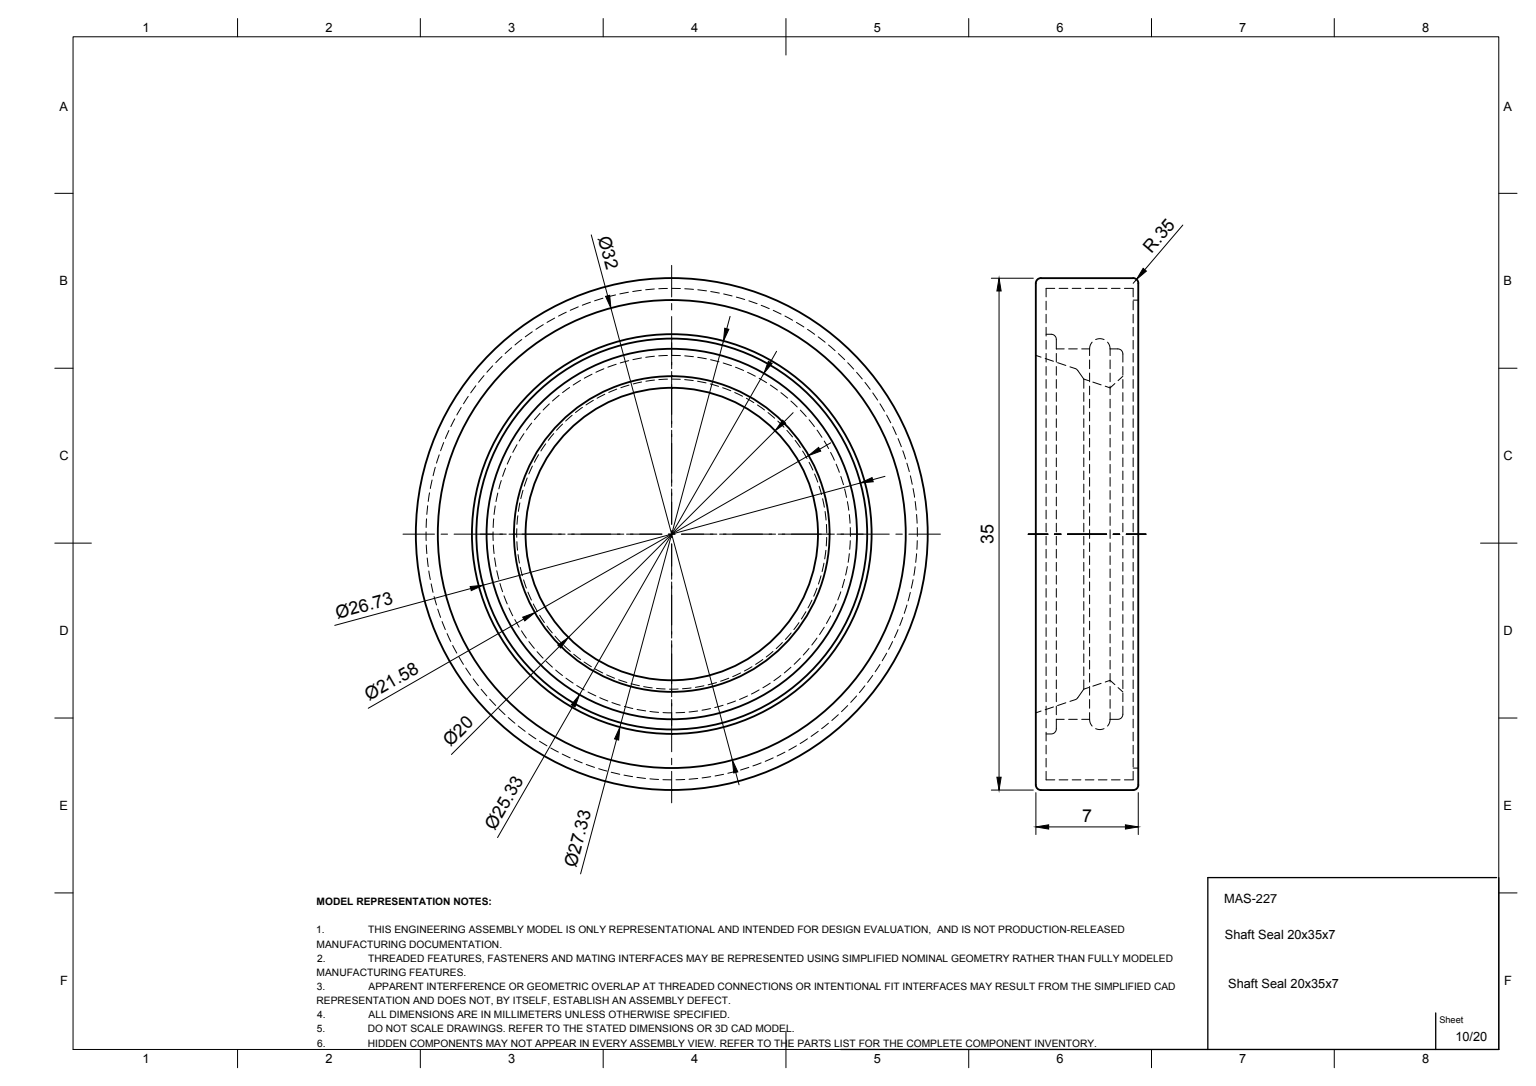
ISO-10303-21;
HEADER;
FILE_DESCRIPTION (('STEP AP214'),
    '1' );
FILE_NAME ( 'Shaft Seal 20x35x7.step', '2026-10-06T08:24:41', ( '' ), ( '' ), 'STEP AP214', 'Unspecified', '' );
FILE_SCHEMA (( 'AUTOMOTIVE_DESIGN' ));
ENDSEC;
DATA;
#55=EDGE_CURVE ( 'NONE', #27011, #13237, #9086, .T. ) ;
#110=CIRCLE ( 'NONE', #17215, 0.4848217985909654137 ) ;
#132=CIRCLE ( 'NONE', #21747, 0.6299212598425196763 ) ;
#156=ORIENTED_EDGE ( 'NONE', *, *, #27125, .T. ) ;
#161=CARTESIAN_POINT ( 'NONE',  ( 0.000000000000000000, 0.000000000000000000, -0.1033464566929133965 ) ) ;
#196=CARTESIAN_POINT ( 'NONE',  ( -0.6751968503937006982, 0.000000000000000000, -0.2618110236220472231 ) ) ;
#313=DIRECTION ( 'NONE',  ( -1.000000000000000000, 0.000000000000000000, 0.000000000000000000 ) ) ;
#322=FACE_OUTER_BOUND ( 'NONE', #12534, .T. ) ;
#345=ORIENTED_EDGE ( 'NONE', *, *, #3993, .T. ) ;
#363=DIRECTION ( 'NONE',  ( 0.000000000000000000, 0.000000000000000000, -1.000000000000000000 ) ) ;
#374=AXIS2_PLACEMENT_3D ( 'NONE', #10936, #6568, #8678 ) ;
#398=DIRECTION ( 'NONE',  ( -1.000000000000000000, 0.000000000000000000, 0.000000000000000000 ) ) ;
#418=DIRECTION ( 'NONE',  ( -1.000000000000000000, 0.000000000000000000, 0.000000000000000000 ) ) ;
#425=AXIS2_PLACEMENT_3D ( 'NONE', #17792, #8636, #2410 ) ;
#446=FACE_BOUND ( 'NONE', #5587, .T. ) ;
#490=CARTESIAN_POINT ( 'NONE',  ( -0.6614173228346456046, 0.000000000000000000, -0.2480314960629921295 ) ) ;
#495=DIRECTION ( 'NONE',  ( 0.000000000000000000, 0.000000000000000000, 1.000000000000000000 ) ) ;
#507=DIRECTION ( 'NONE',  ( 0.000000000000000000, 0.000000000000000000, -1.000000000000000000 ) ) ;
#540=EDGE_LOOP ( 'NONE', ( #5491, #24841, #13223, #6608 ) ) ;
#544=EDGE_CURVE ( 'NONE', #25079, #10563, #9634, .T. ) ;
#545=CIRCLE ( 'NONE', #13618, 0.01377952755905510404 ) ;
#623=CARTESIAN_POINT ( 'NONE',  ( 0.000000000000000000, 0.000000000000000000, -0.05511811023622047168 ) ) ;
#825=EDGE_CURVE ( 'NONE', #24109, #24279, #17361, .T. ) ;
#839=ORIENTED_EDGE ( 'NONE', *, *, #24552, .T. ) ;
#850=AXIS2_PLACEMENT_3D ( 'NONE', #25833, #6763, #15396 ) ;
#877=AXIS2_PLACEMENT_3D ( 'NONE', #9629, #24334, #22215 ) ;
#909=AXIS2_PLACEMENT_3D ( 'NONE', #18396, #16022, #13901 ) ;
#932=CARTESIAN_POINT ( 'NONE',  ( 0.6751968503937006982, 8.353151887884997269E-17, -4.097771653543307347E-17 ) ) ;
#943=DIRECTION ( 'NONE',  ( 1.000000000000000000, 0.000000000000000000, 0.000000000000000000 ) ) ;
#1020=DIRECTION ( 'NONE',  ( -1.000000000000000000, 0.000000000000000000, 0.000000000000000000 ) ) ;
#1062=VECTOR ( 'NONE', #24990, 39.37007874015748143 ) ;
#1129=CARTESIAN_POINT ( 'NONE',  ( -0.5850448763834590338, 0.000000000000000000, -0.2755905511811023723 ) ) ;
#1147=ORIENTED_EDGE ( 'NONE', *, *, #20181, .T. ) ;
#1182=ADVANCED_FACE ( 'NONE', ( #9849 ), #22775, .T. ) ;
#1214=EDGE_LOOP ( 'NONE', ( #23740, #11327, #1147, #4046 ) ) ;
#1232=ORIENTED_EDGE ( 'NONE', *, *, #23960, .F. ) ;
#1257=CARTESIAN_POINT ( 'NONE',  ( -0.4173606904761050229, 0.000000000000000000, -0.1464516454673935042 ) ) ;
#1259=ORIENTED_EDGE ( 'NONE', *, *, #11342, .T. ) ;
#1336=( CONVERSION_BASED_UNIT ( 'INCH', #25059 ) LENGTH_UNIT ( ) NAMED_UNIT ( #10443 ) ) ;
#1337=VECTOR ( 'NONE', #1696, 39.37007874015748854 ) ;
#1355=DIRECTION ( 'NONE',  ( -1.000000000000000000, 0.000000000000000000, 0.000000000000000000 ) ) ;
#1357=ORIENTED_EDGE ( 'NONE', *, *, #3422, .F. ) ;
#1416=EDGE_LOOP ( 'NONE', ( #17196, #23650, #10052, #15549 ) ) ;
#1470=CARTESIAN_POINT ( 'NONE',  ( 0.4848217985909654137, 6.021729909607683004E-17, -0.04133858267716535029 ) ) ;
#1492=AXIS2_PLACEMENT_3D ( 'NONE', #22889, #26835, #7774 ) ;
#1536=AXIS2_PLACEMENT_3D ( 'NONE', #16554, #14463, #7522 ) ;
#1541=CIRCLE ( 'NONE', #24983, 0.6614173228346456046 ) ;
#1574=FACE_OUTER_BOUND ( 'NONE', #540, .T. ) ;
#1603=ORIENTED_EDGE ( 'NONE', *, *, #23444, .F. ) ;
#1619=CARTESIAN_POINT ( 'NONE',  ( 0.5379714048901780288, 6.588249590315613132E-17, -0.2480314960629921295 ) ) ;
#1641=CIRCLE ( 'NONE', #24186, 0.01377952755905510404 ) ;
#1646=LINE ( 'NONE', #27513, #5048 ) ;
#1678=CARTESIAN_POINT ( 'NONE',  ( 0.000000000000000000, 0.000000000000000000, -0.01377952755905511792 ) ) ;
#1696=DIRECTION ( 'NONE',  ( -0.6698894744055998718, 0.000000000000000000, 0.7424608353849979636 ) ) ;
#1697=CARTESIAN_POINT ( 'NONE',  ( 0.5241918773311228241, 6.419499047126015796E-17, -0.2342519685039370358 ) ) ;
#1735=VECTOR ( 'NONE', #24190, 39.37007874015748854 ) ;
#1792=DIRECTION ( 'NONE',  ( -1.000000000000000000, -1.224646799147356165E-16, 0.000000000000000000 ) ) ;
#1807=CARTESIAN_POINT ( 'NONE',  ( 0.6889763779527560139, 8.437527159479796553E-17, -0.2618110236220472231 ) ) ;
#1817=AXIS2_PLACEMENT_3D ( 'NONE', #6481, #17216, #21462 ) ;
#1838=FACE_OUTER_BOUND ( 'NONE', #26109, .T. ) ;
#1863=CIRCLE ( 'NONE', #3660, 0.4811133748141622202 ) ;
#1903=DIRECTION ( 'NONE',  ( 0.000000000000000000, 0.000000000000000000, -1.000000000000000000 ) ) ;
#1924=DIRECTION ( 'NONE',  ( -1.224646799147353207E-16, 1.000000000000000000, 0.000000000000000000 ) ) ;
#1925=DIRECTION ( 'NONE',  ( -1.000000000000000000, 0.000000000000000000, 0.000000000000000000 ) ) ;
#2015=CARTESIAN_POINT ( 'NONE',  ( -0.6299212598425196763, 0.000000000000000000, -4.370956692913385731E-17 ) ) ;
#2027=DIRECTION ( 'NONE',  ( 1.000000000000000000, 0.000000000000000000, 0.000000000000000000 ) ) ;
#2056=CARTESIAN_POINT ( 'NONE',  ( -0.4456396174367268093, -1.277930342114489576E-27, -0.1696422624804970747 ) ) ;
#2082=CARTESIAN_POINT ( 'NONE',  ( -0.6889763779527560139, 0.000000000000000000, -0.01377952755905511792 ) ) ;
#2174=CARTESIAN_POINT ( 'NONE',  ( 0.4986013261500205074, 6.106105181202481056E-17, -0.05511811023622047168 ) ) ;
#2177=LINE ( 'NONE', #19551, #13048 ) ;
#2184=FACE_BOUND ( 'NONE', #13764, .T. ) ;
#2223=VERTEX_POINT ( 'NONE', #14401 ) ;
#2240=CARTESIAN_POINT ( 'NONE',  ( -0.5996943638624113726, 0.000000000000000000, -0.2480314960629921295 ) ) ;
#2244=ORIENTED_EDGE ( 'NONE', *, *, #3504, .T. ) ;
#2262=CARTESIAN_POINT ( 'NONE',  ( 0.000000000000000000, 0.000000000000000000, -0.1309055118110236116 ) ) ;
#2267=CARTESIAN_POINT ( 'NONE',  ( 0.000000000000000000, 0.000000000000000000, -0.07578740157480315376 ) ) ;
#2276=ORIENTED_EDGE ( 'NONE', *, *, #7179, .T. ) ;
#2284=DIRECTION ( 'NONE',  ( 0.000000000000000000, 0.000000000000000000, -1.000000000000000000 ) ) ;
#2373=DIRECTION ( 'NONE',  ( 1.000000000000000000, 0.000000000000000000, 0.000000000000000000 ) ) ;
#2405=CARTESIAN_POINT ( 'NONE',  ( 0.000000000000000000, 0.000000000000000000, -0.2204724409448818867 ) ) ;
#2410=DIRECTION ( 'NONE',  ( 1.000000000000000000, 0.000000000000000000, 0.000000000000000000 ) ) ;
#2422=EDGE_CURVE ( 'NONE', #3726, #27011, #7034, .T. ) ;
#2429=DIRECTION ( 'NONE',  ( -1.000000000000000000, 0.000000000000000000, 0.000000000000000000 ) ) ;
#2432=EDGE_CURVE ( 'NONE', #12340, #4895, #14270, .T. ) ;
#2433=DIRECTION ( 'NONE',  ( -1.000000000000000000, 0.000000000000000000, 0.000000000000000000 ) ) ;
#2487=VERTEX_POINT ( 'NONE', #490 ) ;
#2548=ORIENTED_EDGE ( 'NONE', *, *, #8868, .F. ) ;
#2579=FACE_OUTER_BOUND ( 'NONE', #25724, .T. ) ;
#2580=EDGE_LOOP ( 'NONE', ( #27237, #13937 ) ) ;
#2585=DIRECTION ( 'NONE',  ( 0.000000000000000000, 0.000000000000000000, -1.000000000000000000 ) ) ;
#2604=ADVANCED_FACE ( 'NONE', ( #15156 ), #8024, .T. ) ;
#2633=EDGE_LOOP ( 'NONE', ( #23889, #12887 ) ) ;
#2685=ORIENTED_EDGE ( 'NONE', *, *, #23444, .T. ) ;
#2704=AXIS2_PLACEMENT_3D ( 'NONE', #14804, #21278, #1355 ) ;
#2729=EDGE_CURVE ( 'NONE', #12355, #25409, #17051, .T. ) ;
#2906=FACE_OUTER_BOUND ( 'NONE', #24076, .T. ) ;
#2916=DIRECTION ( 'NONE',  ( 0.000000000000000000, 0.000000000000000000, -1.000000000000000000 ) ) ;
#2923=CIRCLE ( 'NONE', #4729, 0.6614173228346456046 ) ;
#2962=DIRECTION ( 'NONE',  ( -1.000000000000000000, 0.000000000000000000, 0.000000000000000000 ) ) ;
#3008=EDGE_CURVE ( 'NONE', #23052, #25295, #24687, .T. ) ;
#3022=MANIFOLD_SOLID_BREP ( 'Shaft Seal 20x35x7', #25894 ) ;
#3050=DIRECTION ( 'NONE',  ( 1.000000000000000000, 0.000000000000000000, 0.000000000000000000 ) ) ;
#3097=ADVANCED_FACE ( 'NONE', ( #2906 ), #20667, .T. ) ;
#3143=AXIS2_PLACEMENT_3D ( 'NONE', #25557, #10283, #3501 ) ;
#3205=ADVANCED_FACE ( 'NONE', ( #15750 ), #24270, .T. ) ;
#3275=CARTESIAN_POINT ( 'NONE',  ( 0.3937007874015748254, -5.011764252456519698E-17, -0.07578740157480315376 ) ) ;
#3292=( NAMED_UNIT ( * ) PLANE_ANGLE_UNIT ( ) SI_UNIT ( $, .RADIAN. ) ) ;
#3307=DIRECTION ( 'NONE',  ( 0.000000000000000000, 0.000000000000000000, -1.000000000000000000 ) ) ;
#3366=DIRECTION ( 'NONE',  ( -1.000000000000000000, 0.000000000000000000, 0.000000000000000000 ) ) ;
#3382=CARTESIAN_POINT ( 'NONE',  ( 0.000000000000000000, 0.000000000000000000, -0.2204724409448818867 ) ) ;
#3422=EDGE_CURVE ( 'NONE', #18692, #19022, #26099, .T. ) ;
#3424=CARTESIAN_POINT ( 'NONE',  ( 0.000000000000000000, 0.000000000000000000, -0.2342519685039370358 ) ) ;
#3467=CARTESIAN_POINT ( 'NONE',  ( -0.6889763779527560139, 0.000000000000000000, -0.2618110236220472231 ) ) ;
#3501=DIRECTION ( 'NONE',  ( -1.000000000000000000, 0.000000000000000000, 0.000000000000000000 ) ) ;
#3504=EDGE_CURVE ( 'NONE', #23082, #16707, #15586, .T. ) ;
#3524=EDGE_CURVE ( 'NONE', #5922, #27503, #14854, .T. ) ;
#3548=ORIENTED_EDGE ( 'NONE', *, *, #19521, .F. ) ;
#3553=CARTESIAN_POINT ( 'NONE',  ( 0.000000000000000000, 0.000000000000000000, -0.01377952755905511792 ) ) ;
#3558=FACE_OUTER_BOUND ( 'NONE', #10210, .T. ) ;
#3565=CARTESIAN_POINT ( 'NONE',  ( 0.000000000000000000, 0.000000000000000000, -0.2342519685039370358 ) ) ;
#3570=AXIS2_PLACEMENT_3D ( 'NONE', #23741, #14865, #12984 ) ;
#3588=CIRCLE ( 'NONE', #23495, 0.6299212598425196763 ) ;
#3615=LINE ( 'NONE', #12246, #4669 ) ;
#3644=DIRECTION ( 'NONE',  ( 0.000000000000000000, 0.000000000000000000, 1.000000000000000000 ) ) ;
#3660=AXIS2_PLACEMENT_3D ( 'NONE', #26675, #26822, #22446 ) ;
#3665=DIRECTION ( 'NONE',  ( 0.000000000000000000, 0.000000000000000000, 1.000000000000000000 ) ) ;
#3726=VERTEX_POINT ( 'NONE', #24193 ) ;
#3780=ORIENTED_EDGE ( 'NONE', *, *, #20283, .F. ) ;
#3817=AXIS2_PLACEMENT_3D ( 'NONE', #5847, #27177, #7818 ) ;
#3880=AXIS2_PLACEMENT_3D ( 'NONE', #5456, #3307, #11949 ) ;
#3910=EDGE_LOOP ( 'NONE', ( #15781, #1259, #839, #24102 ) ) ;
#3930=CARTESIAN_POINT ( 'NONE',  ( 0.4055307389460929279, 4.966319214061935299E-17, -0.1111195235210984261 ) ) ;
#3978=CIRCLE ( 'NONE', #19758, 0.6889763779527560139 ) ;
#3989=CARTESIAN_POINT ( 'NONE',  ( 0.000000000000000000, 0.000000000000000000, -0.2618110236220472231 ) ) ;
#3993=EDGE_CURVE ( 'NONE', #3726, #15200, #17111, .T. ) ;
#3996=AXIS2_PLACEMENT_3D ( 'NONE', #161, #4361, #418 ) ;
#4046=ORIENTED_EDGE ( 'NONE', *, *, #6905, .F. ) ;
#4062=ORIENTED_EDGE ( 'NONE', *, *, #15737, .F. ) ;
#4084=CIRCLE ( 'NONE', #19402, 0.01377952755905510404 ) ;
#4138=DIRECTION ( 'NONE',  ( -1.000000000000000000, -1.224646799147356165E-16, 0.000000000000000000 ) ) ;
#4222=CARTESIAN_POINT ( 'NONE',  ( -0.4307823082429378392, 0.000000000000000000, -0.1559029880880275776 ) ) ;
#4226=LINE ( 'NONE', #26104, #11288 ) ;
#4256=DIRECTION ( 'NONE',  ( 0.000000000000000000, 0.000000000000000000, -1.000000000000000000 ) ) ;
#4283=LINE ( 'NONE', #9058, #23272 ) ;
#4287=TOROIDAL_SURFACE ( 'NONE', #7899, 0.6751968503937006982, 0.01377952755905511792 ) ;
#4290=EDGE_LOOP ( 'NONE', ( #7597, #11737 ) ) ;
#4345=ORIENTED_EDGE ( 'NONE', *, *, #19521, .T. ) ;
#4361=DIRECTION ( 'NONE',  ( 0.000000000000000000, 0.000000000000000000, -1.000000000000000000 ) ) ;
#4390=CARTESIAN_POINT ( 'NONE',  ( 0.6299212598425196763, 7.714310545810098438E-17, -0.01377952755905511792 ) ) ;
#4401=DIRECTION ( 'NONE',  ( -1.000000000000000000, 0.000000000000000000, 0.000000000000000000 ) ) ;
#4465=EDGE_CURVE ( 'NONE', #24279, #12499, #12727, .T. ) ;
#4470=AXIS2_PLACEMENT_3D ( 'NONE', #9684, #5310, #943 ) ;
#4476=EDGE_LOOP ( 'NONE', ( #27104, #19325, #20943, #13965 ) ) ;
#4480=CIRCLE ( 'NONE', #9406, 0.6751968503937006982 ) ;
#4510=CARTESIAN_POINT ( 'NONE',  ( 0.000000000000000000, 0.000000000000000000, -0.2342519685039370358 ) ) ;
#4538=CARTESIAN_POINT ( 'NONE',  ( 0.4173606904761050229, 5.111194336814911913E-17, -0.1464516454673935042 ) ) ;
#4552=VERTEX_POINT ( 'NONE', #2082 ) ;
#4573=EDGE_CURVE ( 'NONE', #16402, #11118, #26557, .T. ) ;
#4642=CARTESIAN_POINT ( 'NONE',  ( 0.6751968503937006982, 8.353151887884997269E-17, -0.2755905511811023723 ) ) ;
#4669=VECTOR ( 'NONE', #6048, 39.37007874015748143 ) ;
#4729=AXIS2_PLACEMENT_3D ( 'NONE', #14420, #9581, #12972 ) ;
#4743=CARTESIAN_POINT ( 'NONE',  ( 0.000000000000000000, 0.000000000000000000, -0.006889763779527558960 ) ) ;
#4786=EDGE_LOOP ( 'NONE', ( #13307, #18454, #15039, #24615 ) ) ;
#4863=EDGE_LOOP ( 'NONE', ( #16587, #345, #25002, #11154 ) ) ;
#4895=VERTEX_POINT ( 'NONE', #2174 ) ;
#4909=FACE_OUTER_BOUND ( 'NONE', #12771, .T. ) ;
#4947=FACE_OUTER_BOUND ( 'NONE', #10950, .T. ) ;
#5048=VECTOR ( 'NONE', #17907, 39.37007874015748143 ) ;
#5055=ORIENTED_EDGE ( 'NONE', *, *, #15114, .F. ) ;
#5144=ORIENTED_EDGE ( 'NONE', *, *, #2432, .T. ) ;
#5145=CIRCLE ( 'NONE', #3817, 0.5379714048901780288 ) ;
#5158=AXIS2_PLACEMENT_3D ( 'NONE', #4510, #15126, #12978 ) ;
#5229=CARTESIAN_POINT ( 'NONE',  ( 0.000000000000000000, 0.000000000000000000, 0.000000000000000000 ) ) ;
#5235=ORIENTED_EDGE ( 'NONE', *, *, #8944, .T. ) ;
#5239=ADVANCED_FACE ( 'NONE', ( #4947 ), #24748, .F. ) ;
#5281=DIRECTION ( 'NONE',  ( -1.000000000000000000, 0.000000000000000000, 0.000000000000000000 ) ) ;
#5293=ORIENTED_EDGE ( 'NONE', *, *, #21682, .F. ) ;
#5310=DIRECTION ( 'NONE',  ( 0.000000000000000000, 0.000000000000000000, 1.000000000000000000 ) ) ;
#5318=VECTOR ( 'NONE', #11192, 39.37007874015748143 ) ;
#5353=ADVANCED_FACE ( 'NONE', ( #6089, #12977 ), #14853, .T. ) ;
#5358=CARTESIAN_POINT ( 'NONE',  ( 0.000000000000000000, 0.000000000000000000, -0.05511811023622047168 ) ) ;
#5449=CARTESIAN_POINT ( 'NONE',  ( 0.000000000000000000, 0.000000000000000000, -0.04133858267716535029 ) ) ;
#5456=CARTESIAN_POINT ( 'NONE',  ( 0.000000000000000000, 0.000000000000000000, -0.2480314960629921295 ) ) ;
#5464=CARTESIAN_POINT ( 'NONE',  ( 0.000000000000000000, 0.000000000000000000, -0.2204724409448818867 ) ) ;
#5488=ADVANCED_FACE ( 'NONE', ( #4909 ), #13663, .F. ) ;
#5491=ORIENTED_EDGE ( 'NONE', *, *, #544, .T. ) ;
#5587=EDGE_LOOP ( 'NONE', ( #13267, #5293 ) ) ;
#5786=PRODUCT_DEFINITION_FORMATION_WITH_SPECIFIED_SOURCE ( 'ANY', '', #10231, .NOT_KNOWN. ) ;
#5809=DIRECTION ( 'NONE',  ( -1.000000000000000000, -1.224646799147356165E-16, 0.000000000000000000 ) ) ;
#5838=DIRECTION ( 'NONE',  ( 0.000000000000000000, 0.000000000000000000, -1.000000000000000000 ) ) ;
#5847=CARTESIAN_POINT ( 'NONE',  ( 0.000000000000000000, 0.000000000000000000, -0.2342519685039370358 ) ) ;
#5901=DIRECTION ( 'NONE',  ( -1.000000000000000000, 0.000000000000000000, 0.000000000000000000 ) ) ;
#5907=EDGE_CURVE ( 'NONE', #25295, #23039, #2177, .T. ) ;
#5922=VERTEX_POINT ( 'NONE', #1470 ) ;
#6048=DIRECTION ( 'NONE',  ( 0.000000000000000000, 0.000000000000000000, -1.000000000000000000 ) ) ;
#6055=PRODUCT_CONTEXT ( 'NONE', #6560, 'mechanical' ) ;
#6070=ORIENTED_EDGE ( 'NONE', *, *, #14605, .T. ) ;
#6072=CIRCLE ( 'NONE', #1536, 0.6751968503937006982 ) ;
#6089=FACE_BOUND ( 'NONE', #20083, .T. ) ;
#6103=CARTESIAN_POINT ( 'NONE',  ( 0.000000000000000000, 0.000000000000000000, -0.01377952755905511792 ) ) ;
#6125=CARTESIAN_POINT ( 'NONE',  ( -0.6751968503937006982, 0.000000000000000000, -4.097771653543307347E-17 ) ) ;
#6171=LINE ( 'NONE', #21406, #12454 ) ;
#6186=EDGE_CURVE ( 'NONE', #23082, #27011, #26137, .T. ) ;
#6232=CONICAL_SURFACE ( 'NONE', #374, 0.4626586504047134341, 0.3230892413134545116 ) ;
#6264=AXIS2_PLACEMENT_3D ( 'NONE', #12898, #21525, #2027 ) ;
#6273=DIRECTION ( 'NONE',  ( -1.000000000000000000, 0.000000000000000000, 0.000000000000000000 ) ) ;
#6282=PRODUCT_DEFINITION_CONTEXT ( 'detailed design', #13230, 'design' ) ;
#6313=DIRECTION ( 'NONE',  ( -1.000000000000000000, -1.224646799147356165E-16, 0.000000000000000000 ) ) ;
#6322=ORIENTED_EDGE ( 'NONE', *, *, #20618, .T. ) ;
#6362=CARTESIAN_POINT ( 'NONE',  ( -0.4092416079569000109, 0.000000000000000000, -0.05856299212598425896 ) ) ;
#6410=DIRECTION ( 'NONE',  ( 0.000000000000000000, 0.000000000000000000, -1.000000000000000000 ) ) ;
#6423=TOROIDAL_SURFACE ( 'NONE', #16342, 0.5241918773311228241, 0.01377952755905511792 ) ;
#6481=CARTESIAN_POINT ( 'NONE',  ( 0.000000000000000000, 0.000000000000000000, -4.097771653543307347E-17 ) ) ;
#6505=DIRECTION ( 'NONE',  ( 0.000000000000000000, 0.000000000000000000, -1.000000000000000000 ) ) ;
#6521=ADVANCED_FACE ( 'NONE', ( #8833 ), #25698, .F. ) ;
#6523=DIRECTION ( 'NONE',  ( 0.000000000000000000, 0.000000000000000000, -1.000000000000000000 ) ) ;
#6525=CIRCLE ( 'NONE', #19618, 0.6299212598425196763 ) ;
#6539=EDGE_LOOP ( 'NONE', ( #14520, #16363 ) ) ;
#6560=APPLICATION_CONTEXT ( 'automotive_design' ) ;
#6568=DIRECTION ( 'NONE',  ( 0.000000000000000000, 0.000000000000000000, -1.000000000000000000 ) ) ;
#6582=FACE_OUTER_BOUND ( 'NONE', #22443, .T. ) ;
#6608=ORIENTED_EDGE ( 'NONE', *, *, #8944, .F. ) ;
#6622=LINE ( 'NONE', #4222, #7707 ) ;
#6656=CARTESIAN_POINT ( 'NONE',  ( 0.6614173228346456046, 8.100026073100603114E-17, -0.01377952755905511792 ) ) ;
#6670=AXIS2_PLACEMENT_3D ( 'NONE', #21700, #1924, #6313 ) ;
#6687=DIRECTION ( 'NONE',  ( 0.000000000000000000, 0.000000000000000000, -1.000000000000000000 ) ) ;
#6741=FACE_OUTER_BOUND ( 'NONE', #22510, .T. ) ;
#6746=ORIENTED_EDGE ( 'NONE', *, *, #22676, .F. ) ;
#6763=DIRECTION ( 'NONE',  ( 0.000000000000000000, 0.000000000000000000, -1.000000000000000000 ) ) ;
#6765=ORIENTED_EDGE ( 'NONE', *, *, #13241, .T. ) ;
#6844=AXIS2_PLACEMENT_3D ( 'NONE', #15634, #7014, #398 ) ;
#6865=CARTESIAN_POINT ( 'NONE',  ( 0.4811133747915324332, 5.891939544654311124E-17, -0.2755905511811023723 ) ) ;
#6872=DIRECTION ( 'NONE',  ( 0.000000000000000000, 0.000000000000000000, -1.000000000000000000 ) ) ;
#6888=CIRCLE ( 'NONE', #27663, 0.4173606904906118076 ) ;
#6905=EDGE_CURVE ( 'NONE', #15200, #23082, #4084, .T. ) ;
#7014=DIRECTION ( 'NONE',  ( 0.000000000000000000, 0.000000000000000000, -1.000000000000000000 ) ) ;
#7034=CIRCLE ( 'NONE', #26415, 0.01377952755905510404 ) ;
#7043=ADVANCED_FACE ( 'NONE', ( #18761 ), #24810, .F. ) ;
#7064=CIRCLE ( 'NONE', #12020, 0.01377952755905511792 ) ;
#7069=CIRCLE ( 'NONE', #26928, 0.6889763779527560139 ) ;
#7084=EDGE_CURVE ( 'NONE', #4895, #23052, #4226, .T. ) ;
#7087=AXIS2_PLACEMENT_3D ( 'NONE', #21756, #15546, #313 ) ;
#7179=EDGE_CURVE ( 'NONE', #12355, #14847, #8132, .T. ) ;
#7218=ORIENTED_EDGE ( 'NONE', *, *, #24541, .F. ) ;
#7256=DIRECTION ( 'NONE',  ( 1.000000000000000000, 0.000000000000000000, 0.000000000000000000 ) ) ;
#7286=ORIENTED_EDGE ( 'NONE', *, *, #19531, .T. ) ;
#7331=EDGE_CURVE ( 'NONE', #18692, #15200, #6622, .T. ) ;
#7363=ORIENTED_EDGE ( 'NONE', *, *, #12786, .F. ) ;
#7457=SHAPE_REPRESENTATION_RELATIONSHIP ( 'NONE' , 'NONE' ,  #20013, #26510 ) ;
#7461=ORIENTED_EDGE ( 'NONE', *, *, #7084, .T. ) ;
#7474=FACE_OUTER_BOUND ( 'NONE', #18850, .T. ) ;
#7479=EDGE_CURVE ( 'NONE', #10528, #23039, #19417, .T. ) ;
#7522=DIRECTION ( 'NONE',  ( 1.000000000000000000, 0.000000000000000000, 0.000000000000000000 ) ) ;
#7562=DIRECTION ( 'NONE',  ( 0.000000000000000000, 0.000000000000000000, -1.000000000000000000 ) ) ;
#7597=ORIENTED_EDGE ( 'NONE', *, *, #7479, .T. ) ;
#7657=ADVANCED_FACE ( 'NONE', ( #6582 ), #17208, .F. ) ;
#7707=VECTOR ( 'NONE', #15246, 39.37007874015748854 ) ;
#7774=DIRECTION ( 'NONE',  ( 0.000000000000000000, 0.000000000000000000, -1.000000000000000000 ) ) ;
#7778=DIRECTION ( 'NONE',  ( -1.000000000000000000, 0.000000000000000000, 0.000000000000000000 ) ) ;
#7818=DIRECTION ( 'NONE',  ( 1.000000000000000000, 0.000000000000000000, 0.000000000000000000 ) ) ;
#7836=CARTESIAN_POINT ( 'NONE',  ( 0.000000000000000000, 0.000000000000000000, -0.1464516454673935042 ) ) ;
#7861=ORIENTED_EDGE ( 'NONE', *, *, #21916, .T. ) ;
#7899=AXIS2_PLACEMENT_3D ( 'NONE', #8221, #24734, #25160 ) ;
#7904=DIRECTION ( 'NONE',  ( -0.000000000000000000, -1.000000000000000000, -0.000000000000000000 ) ) ;
#7923=DIRECTION ( 'NONE',  ( 1.000000000000000000, 0.000000000000000000, 0.000000000000000000 ) ) ;
#7976=CARTESIAN_POINT ( 'NONE',  ( 0.000000000000000000, 0.000000000000000000, -0.05856299212598425896 ) ) ;
#7989=DIRECTION ( 'NONE',  ( -1.000000000000000000, 0.000000000000000000, 0.000000000000000000 ) ) ;
#8024=CYLINDRICAL_SURFACE ( 'NONE', #27341, 0.6889763779527560139 ) ;
#8082=ORIENTED_EDGE ( 'NONE', *, *, #27125, .F. ) ;
#8132=CIRCLE ( 'NONE', #1817, 0.6751968503937006982 ) ;
#8200=VECTOR ( 'NONE', #13359, 39.37007874015748143 ) ;
#8206=ORIENTED_EDGE ( 'NONE', *, *, #17821, .F. ) ;
#8209=DIRECTION ( 'NONE',  ( -1.000000000000000000, 0.000000000000000000, 0.000000000000000000 ) ) ;
#8213=ORIENTED_EDGE ( 'NONE', *, *, #24514, .T. ) ;
#8221=CARTESIAN_POINT ( 'NONE',  ( 0.000000000000000000, 0.000000000000000000, -0.2618110236220472231 ) ) ;
#8310=ADVANCED_FACE ( 'NONE', ( #9361, #13755 ), #16170, .T. ) ;
#8322=ORIENTED_EDGE ( 'NONE', *, *, #13018, .F. ) ;
#8433=ORIENTED_EDGE ( 'NONE', *, *, #20611, .F. ) ;
#8479=DIRECTION ( 'NONE',  ( -0.000000000000000000, -1.000000000000000000, -0.000000000000000000 ) ) ;
#8499=( GEOMETRIC_REPRESENTATION_CONTEXT ( 3 ) GLOBAL_UNCERTAINTY_ASSIGNED_CONTEXT ( ( #20901 ) ) GLOBAL_UNIT_ASSIGNED_CONTEXT ( ( #1336, #3292, #20966 ) ) REPRESENTATION_CONTEXT ( 'NONE', 'WORKASPACE' ) ) ;
#8588=ORIENTED_EDGE ( 'NONE', *, *, #5907, .T. ) ;
#8634=TOROIDAL_SURFACE ( 'NONE', #6844, 0.4325730547867440712, 0.01377952755905511792 ) ;
#8636=DIRECTION ( 'NONE',  ( 0.000000000000000000, 0.000000000000000000, 1.000000000000000000 ) ) ;
#8650=CARTESIAN_POINT ( 'NONE',  ( 0.000000000000000000, -5.457511811023621697E-17, -0.1696422624804970747 ) ) ;
#8676=EDGE_CURVE ( 'NONE', #12052, #11811, #23099, .T. ) ;
#8678=DIRECTION ( 'NONE',  ( -1.000000000000000000, 0.000000000000000000, 0.000000000000000000 ) ) ;
#8776=EDGE_LOOP ( 'NONE', ( #17052, #12323, #26672, #8433 ) ) ;
#8781=ORIENTED_EDGE ( 'NONE', *, *, #14920, .F. ) ;
#8814=DIRECTION ( 'NONE',  ( 1.000000000000000000, 0.000000000000000000, 0.000000000000000000 ) ) ;
#8833=FACE_OUTER_BOUND ( 'NONE', #4863, .T. ) ;
#8856=AXIS2_PLACEMENT_3D ( 'NONE', #8650, #2284, #8919 ) ;
#8868=EDGE_CURVE ( 'NONE', #16539, #22124, #11026, .T. ) ;
#8898=DIRECTION ( 'NONE',  ( -1.000000000000000000, 0.000000000000000000, 0.000000000000000000 ) ) ;
#8917=EDGE_CURVE ( 'NONE', #13542, #25295, #14073, .T. ) ;
#8919=DIRECTION ( 'NONE',  ( 1.000000000000000000, 0.000000000000000000, 0.000000000000000000 ) ) ;
#8939=TOROIDAL_SURFACE ( 'NONE', #13021, 0.6751968503937006982, 0.01377952755905511792 ) ;
#8944=EDGE_CURVE ( 'NONE', #25079, #2223, #545, .T. ) ;
#8948=CARTESIAN_POINT ( 'NONE',  ( -0.4986013261500205074, 0.000000000000000000, -0.1033464566929133965 ) ) ;
#8951=ORIENTED_EDGE ( 'NONE', *, *, #19728, .F. ) ;
#9054=DIRECTION ( 'NONE',  ( 0.000000000000000000, 0.000000000000000000, -1.000000000000000000 ) ) ;
#9057=EDGE_LOOP ( 'NONE', ( #9907, #2276, #10800, #14077 ) ) ;
#9058=CARTESIAN_POINT ( 'NONE',  ( -0.6614173228346456046, 0.000000000000000000, -0.1309055118110236116 ) ) ;
#9084=ORIENTED_EDGE ( 'NONE', *, *, #22356, .F. ) ;
#9086=LINE ( 'NONE', #17702, #27247 ) ;
#9212=DIRECTION ( 'NONE',  ( 0.000000000000000000, 0.000000000000000000, 1.000000000000000000 ) ) ;
#9223=AXIS2_PLACEMENT_3D ( 'NONE', #14251, #27097, #12249 ) ;
#9256=AXIS2_PLACEMENT_3D ( 'NONE', #8948, #15473, #2585 ) ;
#9295=DIRECTION ( 'NONE',  ( -1.000000000000000000, 0.000000000000000000, 0.000000000000000000 ) ) ;
#9307=DIRECTION ( 'NONE',  ( 0.000000000000000000, 0.000000000000000000, 1.000000000000000000 ) ) ;
#9321=FACE_OUTER_BOUND ( 'NONE', #9057, .T. ) ;
#9326=CARTESIAN_POINT ( 'NONE',  ( 0.000000000000000000, 0.000000000000000000, -0.07578740157480315376 ) ) ;
#9361=FACE_BOUND ( 'NONE', #4290, .T. ) ;
#9406=AXIS2_PLACEMENT_3D ( 'NONE', #27219, #16761, #22695 ) ;
#9459=ORIENTED_EDGE ( 'NONE', *, *, #14408, .F. ) ;
#9520=DIRECTION ( 'NONE',  ( 1.000000000000000000, 0.000000000000000000, 0.000000000000000000 ) ) ;
#9533=CARTESIAN_POINT ( 'NONE',  ( -0.5241918773311228241, 0.000000000000000000, -0.2204724409448818867 ) ) ;
#9581=DIRECTION ( 'NONE',  ( 0.000000000000000000, 0.000000000000000000, -1.000000000000000000 ) ) ;
#9585=UNCERTAINTY_MEASURE_WITH_UNIT (LENGTH_MEASURE( 1.000000000000000082E-05 ), #14261, 'distance_accuracy_value', 'NONE') ;
#9588=CARTESIAN_POINT ( 'NONE',  ( 0.000000000000000000, 0.000000000000000000, -0.01377952755905511792 ) ) ;
#9607=ORIENTED_EDGE ( 'NONE', *, *, #8917, .T. ) ;
#9615=CARTESIAN_POINT ( 'NONE',  ( 0.6889763779527560139, 8.437527159479796553E-17, -0.01377952755905511792 ) ) ;
#9629=CARTESIAN_POINT ( 'NONE',  ( 0.000000000000000000, 0.000000000000000000, -0.07578740157480315376 ) ) ;
#9634=CIRCLE ( 'NONE', #20031, 0.6889763779527560139 ) ;
#9684=CARTESIAN_POINT ( 'NONE',  ( 0.000000000000000000, 0.000000000000000000, -0.2755905511811023723 ) ) ;
#9692=ADVANCED_FACE ( 'NONE', ( #16445 ), #15043, .F. ) ;
#9748=ORIENTED_EDGE ( 'NONE', *, *, #20283, .T. ) ;
#9813=( GEOMETRIC_REPRESENTATION_CONTEXT ( 3 ) GLOBAL_UNCERTAINTY_ASSIGNED_CONTEXT ( ( #9585 ) ) GLOBAL_UNIT_ASSIGNED_CONTEXT ( ( #14261, #18169, #14104 ) ) REPRESENTATION_CONTEXT ( 'NONE', 'WORKASPACE' ) ) ;
#9849=FACE_OUTER_BOUND ( 'NONE', #8776, .T. ) ;
#9851=EDGE_CURVE ( 'NONE', #12340, #27804, #23789, .T. ) ;
#9889=ORIENTED_EDGE ( 'NONE', *, *, #19531, .F. ) ;
#9907=ORIENTED_EDGE ( 'NONE', *, *, #2729, .F. ) ;
#9945=ORIENTED_EDGE ( 'NONE', *, *, #3524, .T. ) ;
#9954=EDGE_LOOP ( 'NONE', ( #20171, #20807, #2244, #7861 ) ) ;
#10000=CARTESIAN_POINT ( 'NONE',  ( 0.000000000000000000, 0.000000000000000000, -0.05511811023622047168 ) ) ;
#10010=EDGE_CURVE ( 'NONE', #23052, #27804, #26739, .T. ) ;
#10027=ORIENTED_EDGE ( 'NONE', *, *, #17078, .T. ) ;
#10052=ORIENTED_EDGE ( 'NONE', *, *, #13853, .T. ) ;
#10078=DIRECTION ( 'NONE',  ( -1.000000000000000000, 0.000000000000000000, 0.000000000000000000 ) ) ;
#10092=DIRECTION ( 'NONE',  ( 0.000000000000000000, 0.000000000000000000, -1.000000000000000000 ) ) ;
#10096=ORIENTED_EDGE ( 'NONE', *, *, #12786, .T. ) ;
#10097=CIRCLE ( 'NONE', #21403, 0.01377952755905510404 ) ;
#10210=EDGE_LOOP ( 'NONE', ( #16575, #7286, #13502, #17625 ) ) ;
#10231=PRODUCT ( 'Shaft Seal 20x35x7', 'Shaft Seal 20x35x7', '', ( #6055 ) ) ;
#10258=ADVANCED_FACE ( 'NONE', ( #16528 ), #27846, .T. ) ;
#10283=DIRECTION ( 'NONE',  ( 0.000000000000000000, 0.000000000000000000, -1.000000000000000000 ) ) ;
#10299=CARTESIAN_POINT ( 'NONE',  ( -0.4405067310592692409, 0.000000000000000000, -0.1627508102905848297 ) ) ;
#10337=PLANE ( 'NONE',  #27093 ) ;
#10371=EDGE_LOOP ( 'NONE', ( #19536, #17742, #7363, #16897 ) ) ;
#10406=ORIENTED_EDGE ( 'NONE', *, *, #3422, .T. ) ;
#10443=DIMENSIONAL_EXPONENTS ( 1.000000000000000000, 0.000000000000000000, 0.000000000000000000, 0.000000000000000000, 0.000000000000000000, 0.000000000000000000, 0.000000000000000000 ) ;
#10528=VERTEX_POINT ( 'NONE', #14696 ) ;
#10547=EDGE_CURVE ( 'NONE', #11118, #19022, #23303, .T. ) ;
#10563=VERTEX_POINT ( 'NONE', #1807 ) ;
#10589=DIRECTION ( 'NONE',  ( -1.000000000000000000, 0.000000000000000000, 0.000000000000000000 ) ) ;
#10649=ADVANCED_FACE ( 'NONE', ( #21992 ), #26225, .F. ) ;
#10768=AXIS2_PLACEMENT_3D ( 'NONE', #16076, #2916, #26652 ) ;
#10800=ORIENTED_EDGE ( 'NONE', *, *, #27340, .T. ) ;
#10858=CARTESIAN_POINT ( 'NONE',  ( 0.4092416079569000109, -5.011764252623336046E-17, -0.05856299212598425896 ) ) ;
#10872=DIRECTION ( 'NONE',  ( 0.000000000000000000, 0.000000000000000000, -1.000000000000000000 ) ) ;
#10906=ORIENTED_EDGE ( 'NONE', *, *, #27340, .F. ) ;
#10936=CARTESIAN_POINT ( 'NONE',  ( 0.000000000000000000, 0.000000000000000000, -0.2204724409448818867 ) ) ;
#10938=CARTESIAN_POINT ( 'NONE',  ( 0.4325730547867440712, 5.297492069419787030E-17, -0.1740172276534823204 ) ) ;
#10950=EDGE_LOOP ( 'NONE', ( #18419, #13501, #8781, #9084 ) ) ;
#10997=DIRECTION ( 'NONE',  ( 0.000000000000000000, 0.000000000000000000, -1.000000000000000000 ) ) ;
#11013=ORIENTED_EDGE ( 'NONE', *, *, #21838, .T. ) ;
#11026=LINE ( 'NONE', #17520, #25341 ) ;
#11066=DIMENSIONAL_EXPONENTS ( 1.000000000000000000, 0.000000000000000000, 0.000000000000000000, 0.000000000000000000, 0.000000000000000000, 0.000000000000000000, 0.000000000000000000 ) ;
#11083=AXIS2_PLACEMENT_3D ( 'NONE', #623, #9212, #22083 ) ;
#11118=VERTEX_POINT ( 'NONE', #3275 ) ;
#11149=AXIS2_PLACEMENT_3D ( 'NONE', #15376, #6872, #17599 ) ;
#11154=ORIENTED_EDGE ( 'NONE', *, *, #6186, .T. ) ;
#11157=AXIS2_PLACEMENT_3D ( 'NONE', #11798, #7562, #13631 ) ;
#11192=DIRECTION ( 'NONE',  ( 0.000000000000000000, 0.000000000000000000, -1.000000000000000000 ) ) ;
#11257=ORIENTED_EDGE ( 'NONE', *, *, #20611, .T. ) ;
#11288=VECTOR ( 'NONE', #19329, 39.37007874015748143 ) ;
#11327=ORIENTED_EDGE ( 'NONE', *, *, #2422, .T. ) ;
#11332=ORIENTED_EDGE ( 'NONE', *, *, #7331, .F. ) ;
#11342=EDGE_CURVE ( 'NONE', #12052, #24279, #21796, .T. ) ;
#11352=ADVANCED_FACE ( 'NONE', ( #17096 ), #15495, .F. ) ;
#11370=AXIS2_PLACEMENT_3D ( 'NONE', #20240, #23472, #14730 ) ;
#11424=CIRCLE ( 'NONE', #27227, 0.4986013261500205074 ) ;
#11588=AXIS2_PLACEMENT_3D ( 'NONE', #5229, #3665, #7923 ) ;
#11625=ORIENTED_EDGE ( 'NONE', *, *, #7331, .T. ) ;
#11653=DIRECTION ( 'NONE',  ( 0.000000000000000000, 0.000000000000000000, -1.000000000000000000 ) ) ;
#11669=CARTESIAN_POINT ( 'NONE',  ( 0.4986013261500205074, 6.106105181202481056E-17, -0.07578740157480315376 ) ) ;
#11727=CARTESIAN_POINT ( 'NONE',  ( -0.4986013261500205074, 0.000000000000000000, -0.07578740157480315376 ) ) ;
#11737=ORIENTED_EDGE ( 'NONE', *, *, #15737, .T. ) ;
#11798=CARTESIAN_POINT ( 'NONE',  ( 0.000000000000000000, 0.000000000000000000, -0.2755905511811023723 ) ) ;
#11811=VERTEX_POINT ( 'NONE', #9533 ) ;
#11850=DIRECTION ( 'NONE',  ( 0.000000000000000000, 0.000000000000000000, -1.000000000000000000 ) ) ;
#11884=ADVANCED_FACE ( 'NONE', ( #27638 ), #16901, .T. ) ;
#11916=ORIENTED_EDGE ( 'NONE', *, *, #3524, .F. ) ;
#11949=DIRECTION ( 'NONE',  ( -1.000000000000000000, 0.000000000000000000, 0.000000000000000000 ) ) ;
#12017=EDGE_LOOP ( 'NONE', ( #2685, #18704, #21995, #8951 ) ) ;
#12020=AXIS2_PLACEMENT_3D ( 'NONE', #22097, #21693, #26460 ) ;
#12045=CYLINDRICAL_SURFACE ( 'NONE', #3570, 0.4986013261500205074 ) ;
#12052=VERTEX_POINT ( 'NONE', #23503 ) ;
#12066=DIRECTION ( 'NONE',  ( 0.000000000000000000, 0.000000000000000000, -1.000000000000000000 ) ) ;
#12088=ADVANCED_FACE ( 'NONE', ( #26118, #25464 ), #10337, .T. ) ;
#12103=AXIS2_PLACEMENT_3D ( 'NONE', #18931, #27566, #8209 ) ;
#12120=DIRECTION ( 'NONE',  ( 1.000000000000000000, 0.000000000000000000, 0.000000000000000000 ) ) ;
#12189=CYLINDRICAL_SURFACE ( 'NONE', #17919, 0.6889763779527560139 ) ;
#12200=CARTESIAN_POINT ( 'NONE',  ( 0.5379714048901780288, 6.588249590315613132E-17, -0.2342519685039370358 ) ) ;
#12246=CARTESIAN_POINT ( 'NONE',  ( -0.4986013261500205074, 0.000000000000000000, -0.1756889763779527769 ) ) ;
#12249=DIRECTION ( 'NONE',  ( -1.000000000000000000, 0.000000000000000000, 0.000000000000000000 ) ) ;
#12323=ORIENTED_EDGE ( 'NONE', *, *, #10010, .T. ) ;
#12340=VERTEX_POINT ( 'NONE', #22820 ) ;
#12346=FILL_AREA_STYLE_COLOUR ( '', #19749 ) ;
#12355=VERTEX_POINT ( 'NONE', #932 ) ;
#12386=DIRECTION ( 'NONE',  ( 1.000000000000000000, 0.000000000000000000, 0.000000000000000000 ) ) ;
#12390=DIRECTION ( 'NONE',  ( 0.000000000000000000, 0.000000000000000000, -1.000000000000000000 ) ) ;
#12420=EDGE_CURVE ( 'NONE', #27503, #5922, #110, .T. ) ;
#12435=DIRECTION ( 'NONE',  ( 0.000000000000000000, 0.000000000000000000, -1.000000000000000000 ) ) ;
#12436=EDGE_LOOP ( 'NONE', ( #23384, #1357, #11625, #18274 ) ) ;
#12454=VECTOR ( 'NONE', #1903, 39.37007874015748143 ) ;
#12479=CARTESIAN_POINT ( 'NONE',  ( 0.000000000000000000, 0.000000000000000000, -4.370956692913385731E-17 ) ) ;
#12499=VERTEX_POINT ( 'NONE', #1619 ) ;
#12512=ORIENTED_EDGE ( 'NONE', *, *, #14408, .T. ) ;
#12534=EDGE_LOOP ( 'NONE', ( #21978, #25205 ) ) ;
#12546=DIRECTION ( 'NONE',  ( 0.3174974722037089969, 3.888222630716479561E-17, -0.9482591181445370054 ) ) ;
#12582=CARTESIAN_POINT ( 'NONE',  ( 0.6299212598425196763, 7.714310545810098438E-17, -4.370956692913385731E-17 ) ) ;
#12589=AXIS2_PLACEMENT_3D ( 'NONE', #2240, #23872, #3050 ) ;
#12600=ADVANCED_FACE ( 'NONE', ( #22964 ), #13148, .T. ) ;
#12651=VERTEX_POINT ( 'NONE', #12773 ) ;
#12654=DIRECTION ( 'NONE',  ( -1.000000000000000000, 0.000000000000000000, 0.000000000000000000 ) ) ;
#12727=LINE ( 'NONE', #12200, #5318 ) ;
#12760=EDGE_LOOP ( 'NONE', ( #1232, #21202 ) ) ;
#12765=EDGE_CURVE ( 'NONE', #21578, #15239, #132, .T. ) ;
#12771=EDGE_LOOP ( 'NONE', ( #18940, #6070, #17357, #8322 ) ) ;
#12773=CARTESIAN_POINT ( 'NONE',  ( 0.4247824284860164945, -5.202084413794395869E-17, -0.04133858267716535029 ) ) ;
#12775=FACE_OUTER_BOUND ( 'NONE', #2580, .T. ) ;
#12786=EDGE_CURVE ( 'NONE', #18597, #12499, #14576, .T. ) ;
#12795=EDGE_CURVE ( 'NONE', #10563, #25079, #15010, .T. ) ;
#12863=CARTESIAN_POINT ( 'NONE',  ( -0.4247824284860164945, 0.000000000000000000, -0.04133858267716535029 ) ) ;
#12887=ORIENTED_EDGE ( 'NONE', *, *, #12765, .F. ) ;
#12898=CARTESIAN_POINT ( 'NONE',  ( 0.000000000000000000, 0.000000000000000000, -0.04133858267716535029 ) ) ;
#12912=PLANE ( 'NONE',  #27871 ) ;
#12972=DIRECTION ( 'NONE',  ( -1.000000000000000000, 0.000000000000000000, 0.000000000000000000 ) ) ;
#12973=LINE ( 'NONE', #10858, #15072 ) ;
#12977=FACE_OUTER_BOUND ( 'NONE', #20455, .T. ) ;
#12978=DIRECTION ( 'NONE',  ( 1.000000000000000000, 0.000000000000000000, 0.000000000000000000 ) ) ;
#12984=DIRECTION ( 'NONE',  ( -1.000000000000000000, 0.000000000000000000, 0.000000000000000000 ) ) ;
#12995=ADVANCED_FACE ( 'NONE', ( #18732 ), #6423, .T. ) ;
#13018=EDGE_CURVE ( 'NONE', #16237, #15239, #1646, .T. ) ;
#13021=AXIS2_PLACEMENT_3D ( 'NONE', #19330, #10997, #27820 ) ;
#13048=VECTOR ( 'NONE', #21673, 39.37007874015748143 ) ;
#13057=CARTESIAN_POINT ( 'NONE',  ( -0.6594488188976378451, 0.000000000000000000, -3.993519685039370632E-17 ) ) ;
#13137=DIRECTION ( 'NONE',  ( 0.000000000000000000, 0.000000000000000000, -1.000000000000000000 ) ) ;
#13148=TOROIDAL_SURFACE ( 'NONE', #26236, 0.4848217985909654137, 0.01377952755905511792 ) ;
#13223=ORIENTED_EDGE ( 'NONE', *, *, #18285, .T. ) ;
#13227=CIRCLE ( 'NONE', #20449, 0.4986013261500205074 ) ;
#13230=APPLICATION_CONTEXT ( 'automotive_design' ) ;
#13237=VERTEX_POINT ( 'NONE', #6865 ) ;
#13241=EDGE_CURVE ( 'NONE', #19022, #18692, #6888, .T. ) ;
#13252=AXIS2_PLACEMENT_3D ( 'NONE', #27367, #14382, #12386 ) ;
#13267=ORIENTED_EDGE ( 'NONE', *, *, #21916, .F. ) ;
#13269=CIRCLE ( 'NONE', #14652, 0.4247824285122252519 ) ;
#13289=CARTESIAN_POINT ( 'NONE',  ( 0.000000000000000000, 0.000000000000000000, -0.04133858267716535029 ) ) ;
#13307=ORIENTED_EDGE ( 'NONE', *, *, #7084, .F. ) ;
#13309=DIRECTION ( 'NONE',  ( 0.000000000000000000, 0.000000000000000000, -1.000000000000000000 ) ) ;
#13359=DIRECTION ( 'NONE',  ( 0.000000000000000000, 0.000000000000000000, -1.000000000000000000 ) ) ;
#13485=EDGE_LOOP ( 'NONE', ( #23366, #11916 ) ) ;
#13501=ORIENTED_EDGE ( 'NONE', *, *, #23784, .T. ) ;
#13502=ORIENTED_EDGE ( 'NONE', *, *, #544, .F. ) ;
#13541=CARTESIAN_POINT ( 'NONE',  ( -0.4811133747915324332, 0.000000000000000000, -0.2755905511811023723 ) ) ;
#13542=VERTEX_POINT ( 'NONE', #15016 ) ;
#13549=ORIENTED_EDGE ( 'NONE', *, *, #26870, .T. ) ;
#13560=CARTESIAN_POINT ( 'NONE',  ( 0.000000000000000000, 0.000000000000000000, -0.05856299212598425896 ) ) ;
#13618=AXIS2_PLACEMENT_3D ( 'NONE', #196, #15285, #23896 ) ;
#13631=DIRECTION ( 'NONE',  ( -1.000000000000000000, 0.000000000000000000, 0.000000000000000000 ) ) ;
#13661=CIRCLE ( 'NONE', #1492, 0.01377952755905510404 ) ;
#13663=CYLINDRICAL_SURFACE ( 'NONE', #10768, 0.6299212598425196763 ) ;
#13722=ORIENTED_EDGE ( 'NONE', *, *, #4465, .F. ) ;
#13754=FACE_BOUND ( 'NONE', #2633, .T. ) ;
#13755=FACE_OUTER_BOUND ( 'NONE', #12760, .T. ) ;
#13764=EDGE_LOOP ( 'NONE', ( #24113, #10027 ) ) ;
#13797=EDGE_CURVE ( 'NONE', #24109, #18597, #26981, .T. ) ;
#13833=VECTOR ( 'NONE', #21170, 39.37007874015748143 ) ;
#13853=EDGE_CURVE ( 'NONE', #11811, #24109, #13661, .T. ) ;
#13883=DIRECTION ( 'NONE',  ( 0.000000000000000000, 0.000000000000000000, -1.000000000000000000 ) ) ;
#13901=DIRECTION ( 'NONE',  ( 0.000000000000000000, -1.000000000000000000, 0.000000000000000000 ) ) ;
#13916=AXIS2_PLACEMENT_3D ( 'NONE', #7836, #6687, #2433 ) ;
#13937=ORIENTED_EDGE ( 'NONE', *, *, #7179, .F. ) ;
#13965=ORIENTED_EDGE ( 'NONE', *, *, #26870, .F. ) ;
#13979=ORIENTED_EDGE ( 'NONE', *, *, #16234, .T. ) ;
#14053=SURFACE_STYLE_USAGE ( .BOTH. , #20820 ) ;
#14073=CIRCLE ( 'NONE', #17667, 0.4986013261500205074 ) ;
#14077=ORIENTED_EDGE ( 'NONE', *, *, #17821, .T. ) ;
#14082=CARTESIAN_POINT ( 'NONE',  ( 0.000000000000000000, 0.000000000000000000, -0.2618110236220472231 ) ) ;
#14104=( NAMED_UNIT ( * ) SI_UNIT ( $, .STERADIAN. ) SOLID_ANGLE_UNIT ( ) ) ;
#14150=AXIS2_PLACEMENT_3D ( 'NONE', #13289, #21772, #4401 ) ;
#14155=DIRECTION ( 'NONE',  ( 0.000000000000000000, 0.000000000000000000, -1.000000000000000000 ) ) ;
#14186=ORIENTED_EDGE ( 'NONE', *, *, #12795, .F. ) ;
#14251=CARTESIAN_POINT ( 'NONE',  ( 0.000000000000000000, 0.000000000000000000, -0.1033464566929133965 ) ) ;
#14261=( CONVERSION_BASED_UNIT ( 'INCH', #26811 ) LENGTH_UNIT ( ) NAMED_UNIT ( #11066 ) ) ;
#14270=CIRCLE ( 'NONE', #11083, 0.4986013261500205074 ) ;
#14288=CIRCLE ( 'NONE', #15717, 0.6299212598425196763 ) ;
#14320=DIRECTION ( 'NONE',  ( -1.000000000000000000, 0.000000000000000000, 0.000000000000000000 ) ) ;
#14381=CARTESIAN_POINT ( 'NONE',  ( 0.000000000000000000, 0.000000000000000000, -0.2342519685039370358 ) ) ;
#14382=DIRECTION ( 'NONE',  ( 0.000000000000000000, 0.000000000000000000, -1.000000000000000000 ) ) ;
#14401=CARTESIAN_POINT ( 'NONE',  ( -0.6751968503937006982, 0.000000000000000000, -0.2755905511811023723 ) ) ;
#14408=EDGE_CURVE ( 'NONE', #13542, #10528, #3615, .T. ) ;
#14418=EDGE_CURVE ( 'NONE', #5922, #4895, #10097, .T. ) ;
#14420=CARTESIAN_POINT ( 'NONE',  ( 0.000000000000000000, 0.000000000000000000, -0.2480314960629921295 ) ) ;
#14440=CARTESIAN_POINT ( 'NONE',  ( 0.000000000000000000, 0.000000000000000000, -0.2342519685039370358 ) ) ;
#14463=DIRECTION ( 'NONE',  ( 0.000000000000000000, 0.000000000000000000, -1.000000000000000000 ) ) ;
#14506=ORIENTED_EDGE ( 'NONE', *, *, #22356, .T. ) ;
#14520=ORIENTED_EDGE ( 'NONE', *, *, #14920, .T. ) ;
#14527=CARTESIAN_POINT ( 'NONE',  ( 0.000000000000000000, 0.000000000000000000, -0.05856299212598425896 ) ) ;
#14536=CARTESIAN_POINT ( 'NONE',  ( 0.4848217985909654137, 5.937354638012884952E-17, -0.05511811023622047168 ) ) ;
#14561=CARTESIAN_POINT ( 'NONE',  ( -0.4055307389460929279, 0.000000000000000000, -0.1111195235210984261 ) ) ;
#14569=VECTOR ( 'NONE', #12546, 39.37007874015748143 ) ;
#14576=CIRCLE ( 'NONE', #11370, 0.5379714048901780288 ) ;
#14605=EDGE_CURVE ( 'NONE', #20499, #21578, #22925, .T. ) ;
#14652=AXIS2_PLACEMENT_3D ( 'NONE', #15305, #15698, #26547 ) ;
#14667=DIRECTION ( 'NONE',  ( -1.000000000000000000, 0.000000000000000000, 0.000000000000000000 ) ) ;
#14696=CARTESIAN_POINT ( 'NONE',  ( -0.4986013261500205074, 0.000000000000000000, -0.2204724409448818867 ) ) ;
#14730=DIRECTION ( 'NONE',  ( -1.000000000000000000, 0.000000000000000000, 0.000000000000000000 ) ) ;
#14733=DIRECTION ( 'NONE',  ( 0.000000000000000000, 0.000000000000000000, -1.000000000000000000 ) ) ;
#14749=CIRCLE ( 'NONE', #3880, 0.6614173228346456046 ) ;
#14761=EDGE_CURVE ( 'NONE', #14847, #12355, #6072, .T. ) ;
#14804=CARTESIAN_POINT ( 'NONE',  ( 0.000000000000000000, 0.000000000000000000, -0.05856299212598425896 ) ) ;
#14835=ORIENTED_EDGE ( 'NONE', *, *, #10547, .T. ) ;
#14847=VERTEX_POINT ( 'NONE', #6125 ) ;
#14853=PLANE ( 'NONE',  #12589 ) ;
#14854=CIRCLE ( 'NONE', #6264, 0.4848217985909654137 ) ;
#14856=CARTESIAN_POINT ( 'NONE',  ( -0.6299212598425196763, 0.000000000000000000, -0.01377952755905511792 ) ) ;
#14861=CARTESIAN_POINT ( 'NONE',  ( 0.000000000000000000, 0.000000000000000000, -0.2618110236220472231 ) ) ;
#14865=DIRECTION ( 'NONE',  ( 0.000000000000000000, 0.000000000000000000, -1.000000000000000000 ) ) ;
#14920=EDGE_CURVE ( 'NONE', #25917, #12651, #13269, .T. ) ;
#14925=CARTESIAN_POINT ( 'NONE',  ( 0.6614173228346456046, 8.100026073100603114E-17, -0.2480314960629921295 ) ) ;
#14940=DIRECTION ( 'NONE',  ( 0.000000000000000000, 0.000000000000000000, -1.000000000000000000 ) ) ;
#14947=AXIS2_PLACEMENT_3D ( 'NONE', #5464, #20992, #14667 ) ;
#15010=CIRCLE ( 'NONE', #16812, 0.6889763779527560139 ) ;
#15016=CARTESIAN_POINT ( 'NONE',  ( -0.4986013261500205074, 0.000000000000000000, -0.1309055118110236116 ) ) ;
#15025=AXIS2_PLACEMENT_3D ( 'NONE', #4743, #15511, #24242 ) ;
#15039=ORIENTED_EDGE ( 'NONE', *, *, #9851, .T. ) ;
#15043=CONICAL_SURFACE ( 'NONE', #20417, 0.4092416079569000109, 0.7340599135827593491 ) ;
#15072=VECTOR ( 'NONE', #26110, 39.37007874015748854 ) ;
#15114=EDGE_CURVE ( 'NONE', #16237, #20499, #6525, .T. ) ;
#15126=DIRECTION ( 'NONE',  ( 0.000000000000000000, 0.000000000000000000, 1.000000000000000000 ) ) ;
#15156=FACE_OUTER_BOUND ( 'NONE', #17028, .T. ) ;
#15170=CARTESIAN_POINT ( 'NONE',  ( 0.6751968503937006982, 8.268776616290199217E-17, -0.2618110236220472231 ) ) ;
#15178=DIRECTION ( 'NONE',  ( 0.000000000000000000, 0.000000000000000000, -1.000000000000000000 ) ) ;
#15200=VERTEX_POINT ( 'NONE', #10299 ) ;
#15226=LINE ( 'NONE', #17729, #8200 ) ;
#15239=VERTEX_POINT ( 'NONE', #14856 ) ;
#15246=DIRECTION ( 'NONE',  ( -0.8176200022776350940, 0.000000000000000000, -0.5757582234545329802 ) ) ;
#15285=DIRECTION ( 'NONE',  ( -0.000000000000000000, -1.000000000000000000, -0.000000000000000000 ) ) ;
#15295=DIRECTION ( 'NONE',  ( -1.000000000000000000, 0.000000000000000000, 0.000000000000000000 ) ) ;
#15305=CARTESIAN_POINT ( 'NONE',  ( 0.000000000000000000, 0.000000000000000000, -0.04133858267716535029 ) ) ;
#15309=ORIENTED_EDGE ( 'NONE', *, *, #5907, .F. ) ;
#15316=DIRECTION ( 'NONE',  ( -1.224646799147353207E-16, 1.000000000000000000, 0.000000000000000000 ) ) ;
#15353=ORIENTED_EDGE ( 'NONE', *, *, #14418, .F. ) ;
#15364=DIRECTION ( 'NONE',  ( -1.000000000000000000, 0.000000000000000000, 0.000000000000000000 ) ) ;
#15376=CARTESIAN_POINT ( 'NONE',  ( 0.000000000000000000, 0.000000000000000000, -0.1309055118110236116 ) ) ;
#15393=EDGE_LOOP ( 'NONE', ( #26059, #22263, #156, #10406 ) ) ;
#15396=DIRECTION ( 'NONE',  ( -1.000000000000000000, 0.000000000000000000, 0.000000000000000000 ) ) ;
#15473=DIRECTION ( 'NONE',  ( -0.000000000000000000, -1.000000000000000000, -0.000000000000000000 ) ) ;
#15492=ORIENTED_EDGE ( 'NONE', *, *, #13797, .T. ) ;
#15493=DIRECTION ( 'NONE',  ( -1.000000000000000000, 0.000000000000000000, 0.000000000000000000 ) ) ;
#15495=CONICAL_SURFACE ( 'NONE', #16844, 0.4055307389460929279, 0.3230892413134540120 ) ;
#15511=DIRECTION ( 'NONE',  ( 0.000000000000000000, 0.000000000000000000, -1.000000000000000000 ) ) ;
#15546=DIRECTION ( 'NONE',  ( 0.000000000000000000, 0.000000000000000000, -1.000000000000000000 ) ) ;
#15547=CARTESIAN_POINT ( 'NONE',  ( 0.4456396174367268093, 5.674725427529967790E-17, -0.1696422624804970747 ) ) ;
#15549=ORIENTED_EDGE ( 'NONE', *, *, #825, .T. ) ;
#15586=LINE ( 'NONE', #19541, #1735 ) ;
#15624=CARTESIAN_POINT ( 'NONE',  ( 0.4986013261500205074, 6.106105181202481056E-17, -0.1309055118110236116 ) ) ;
#15634=CARTESIAN_POINT ( 'NONE',  ( 0.000000000000000000, 0.000000000000000000, -0.1740172276534823204 ) ) ;
#15643=ADVANCED_FACE ( 'NONE', ( #26417 ), #23834, .T. ) ;
#15698=DIRECTION ( 'NONE',  ( 0.000000000000000000, 0.000000000000000000, -1.000000000000000000 ) ) ;
#15708=TOROIDAL_SURFACE ( 'NONE', #16154, 0.4848217985909654137, 0.01377952755905511792 ) ;
#15717=AXIS2_PLACEMENT_3D ( 'NONE', #6103, #6505, #10589 ) ;
#15734=CARTESIAN_POINT ( 'NONE',  ( 0.000000000000000000, 0.000000000000000000, -0.01377952755905511792 ) ) ;
#15737=EDGE_CURVE ( 'NONE', #23039, #10528, #20972, .T. ) ;
#15750=FACE_OUTER_BOUND ( 'NONE', #1416, .T. ) ;
#15781=ORIENTED_EDGE ( 'NONE', *, *, #23960, .T. ) ;
#15835=CARTESIAN_POINT ( 'NONE',  ( 0.000000000000000000, 0.000000000000000000, -0.01377952755905511792 ) ) ;
#15839=AXIS2_PLACEMENT_3D ( 'NONE', #17966, #24766, #7256 ) ;
#15867=ORIENTED_EDGE ( 'NONE', *, *, #825, .F. ) ;
#15954=CIRCLE ( 'NONE', #14150, 0.4247824285122252519 ) ;
#15971=DIRECTION ( 'NONE',  ( 0.000000000000000000, 0.000000000000000000, -1.000000000000000000 ) ) ;
#15993=ORIENTED_EDGE ( 'NONE', *, *, #20181, .F. ) ;
#16022=DIRECTION ( 'NONE',  ( 0.000000000000000000, 0.000000000000000000, -1.000000000000000000 ) ) ;
#16076=CARTESIAN_POINT ( 'NONE',  ( 0.000000000000000000, 0.000000000000000000, -0.006889763779527558960 ) ) ;
#16102=DIRECTION ( 'NONE',  ( 0.000000000000000000, -1.000000000000000000, 0.000000000000000000 ) ) ;
#16140=AXIS2_PLACEMENT_3D ( 'NONE', #20683, #22952, #18686 ) ;
#16154=AXIS2_PLACEMENT_3D ( 'NONE', #5358, #26402, #9295 ) ;
#16170=PLANE ( 'NONE',  #15839 ) ;
#16234=EDGE_CURVE ( 'NONE', #26492, #2487, #4283, .T. ) ;
#16237=VERTEX_POINT ( 'NONE', #2015 ) ;
#16314=SURFACE_STYLE_FILL_AREA ( #25339 ) ;
#16342=AXIS2_PLACEMENT_3D ( 'NONE', #14381, #18579, #5901 ) ;
#16363=ORIENTED_EDGE ( 'NONE', *, *, #23404, .T. ) ;
#16384=ADVANCED_FACE ( 'NONE', ( #9321 ), #25726, .T. ) ;
#16402=VERTEX_POINT ( 'NONE', #27281 ) ;
#16435=CARTESIAN_POINT ( 'NONE',  ( -0.4848217985909654137, 0.000000000000000000, -0.04133858267716535029 ) ) ;
#16437=AXIS2_PLACEMENT_3D ( 'NONE', #3553, #21087, #14320 ) ;
#16445=FACE_OUTER_BOUND ( 'NONE', #25831, .T. ) ;
#16528=FACE_OUTER_BOUND ( 'NONE', #10371, .T. ) ;
#16539=VERTEX_POINT ( 'NONE', #6656 ) ;
#16554=CARTESIAN_POINT ( 'NONE',  ( 0.000000000000000000, 0.000000000000000000, -4.097771653543307347E-17 ) ) ;
#16571=STYLED_ITEM ( 'NONE', ( #23094 ), #3022 ) ;
#16572=CARTESIAN_POINT ( 'NONE',  ( 0.000000000000000000, 0.000000000000000000, -0.07578740157480315376 ) ) ;
#16575=ORIENTED_EDGE ( 'NONE', *, *, #18802, .F. ) ;
#16587=ORIENTED_EDGE ( 'NONE', *, *, #2422, .F. ) ;
#16638=TOROIDAL_SURFACE ( 'NONE', #3996, 0.4986013261500205074, 0.02755905511811023584 ) ;
#16651=ORIENTED_EDGE ( 'NONE', *, *, #21682, .T. ) ;
#16707=VERTEX_POINT ( 'NONE', #13541 ) ;
#16761=DIRECTION ( 'NONE',  ( 0.000000000000000000, 0.000000000000000000, 1.000000000000000000 ) ) ;
#16812=AXIS2_PLACEMENT_3D ( 'NONE', #14861, #12435, #25430 ) ;
#16830=DIRECTION ( 'NONE',  ( 0.000000000000000000, 0.000000000000000000, -1.000000000000000000 ) ) ;
#16844=AXIS2_PLACEMENT_3D ( 'NONE', #18927, #14733, #23338 ) ;
#16889=EDGE_LOOP ( 'NONE', ( #6746, #7461, #1603, #27127 ) ) ;
#16897=ORIENTED_EDGE ( 'NONE', *, *, #13797, .F. ) ;
#16899=ORIENTED_EDGE ( 'NONE', *, *, #16234, .F. ) ;
#16901=CYLINDRICAL_SURFACE ( 'NONE', #2704, 0.4986013261500205074 ) ;
#16928=ORIENTED_EDGE ( 'NONE', *, *, #20172, .F. ) ;
#16945=DIRECTION ( 'NONE',  ( 1.000000000000000000, 0.000000000000000000, 0.000000000000000000 ) ) ;
#16970=ORIENTED_EDGE ( 'NONE', *, *, #2729, .T. ) ;
#17008=ADVANCED_FACE ( 'NONE', ( #13754, #18098 ), #26744, .T. ) ;
#17019=ORIENTED_EDGE ( 'NONE', *, *, #20768, .T. ) ;
#17028=EDGE_LOOP ( 'NONE', ( #9889, #8206, #11013, #14186 ) ) ;
#17042=CARTESIAN_POINT ( 'NONE',  ( 0.000000000000000000, 0.000000000000000000, -0.1559029880880275776 ) ) ;
#17051=CIRCLE ( 'NONE', #6670, 0.01377952755905510404 ) ;
#17052=ORIENTED_EDGE ( 'NONE', *, *, #3008, .F. ) ;
#17069=EDGE_CURVE ( 'NONE', #11118, #16402, #23924, .T. ) ;
#17078=EDGE_CURVE ( 'NONE', #20499, #16237, #3588, .T. ) ;
#17096=FACE_OUTER_BOUND ( 'NONE', #26329, .T. ) ;
#17111=CIRCLE ( 'NONE', #425, 0.4405067310818653881 ) ;
#17132=CARTESIAN_POINT ( 'NONE',  ( 0.000000000000000000, 0.000000000000000000, -0.2480314960629921295 ) ) ;
#17160=DIRECTION ( 'NONE',  ( -1.000000000000000000, 0.000000000000000000, 0.000000000000000000 ) ) ;
#17196=ORIENTED_EDGE ( 'NONE', *, *, #11342, .F. ) ;
#17208=CONICAL_SURFACE ( 'NONE', #22150, 0.4307823082429378392, 0.9572651268756555698 ) ;
#17209=LINE ( 'NONE', #14561, #13833 ) ;
#17215=AXIS2_PLACEMENT_3D ( 'NONE', #5449, #11653, #9520 ) ;
#17216=DIRECTION ( 'NONE',  ( 0.000000000000000000, 0.000000000000000000, -1.000000000000000000 ) ) ;
#17354=CIRCLE ( 'NONE', #24547, 0.4405067310818653881 ) ;
#17357=ORIENTED_EDGE ( 'NONE', *, *, #12765, .T. ) ;
#17361=CIRCLE ( 'NONE', #5158, 0.5379714048901780288 ) ;
#17368=AXIS2_PLACEMENT_3D ( 'NONE', #2405, #6523, #19661 ) ;
#17420=AXIS2_PLACEMENT_3D ( 'NONE', #21619, #8479, #10872 ) ;
#17457=CARTESIAN_POINT ( 'NONE',  ( 0.000000000000000000, 0.000000000000000000, -0.1740172276534823204 ) ) ;
#17469=CIRCLE ( 'NONE', #11157, 0.4811133748141622202 ) ;
#17520=CARTESIAN_POINT ( 'NONE',  ( 0.6614173228346456046, 8.100026073100603114E-17, -0.1309055118110236116 ) ) ;
#17599=DIRECTION ( 'NONE',  ( -1.000000000000000000, 0.000000000000000000, 0.000000000000000000 ) ) ;
#17625=ORIENTED_EDGE ( 'NONE', *, *, #21838, .F. ) ;
#17663=ADVANCED_FACE ( 'NONE', ( #446, #322 ), #24556, .T. ) ;
#17667=AXIS2_PLACEMENT_3D ( 'NONE', #2262, #4256, #8898 ) ;
#17672=DIRECTION ( 'NONE',  ( 0.000000000000000000, 0.000000000000000000, -1.000000000000000000 ) ) ;
#17702=CARTESIAN_POINT ( 'NONE',  ( 0.4626586504047134341, 5.665934353159666004E-17, -0.2204724409448818867 ) ) ;
#17729=CARTESIAN_POINT ( 'NONE',  ( -0.6889763779527560139, 0.000000000000000000, -0.1377952755905511861 ) ) ;
#17742=ORIENTED_EDGE ( 'NONE', *, *, #4465, .T. ) ;
#17768=( LENGTH_UNIT ( ) NAMED_UNIT ( * ) SI_UNIT ( $, .METRE. ) ) ;
#17792=CARTESIAN_POINT ( 'NONE',  ( 0.000000000000000000, -5.394653543307086438E-17, -0.1627508102905848297 ) ) ;
#17794=AXIS2_PLACEMENT_3D ( 'NONE', #14527, #23130, #1925 ) ;
#17797=ADVANCED_FACE ( 'NONE', ( #7474 ), #15708, .T. ) ;
#17821=EDGE_CURVE ( 'NONE', #4552, #25409, #3978, .T. ) ;
#17823=DIRECTION ( 'NONE',  ( 0.3174974722037094410, 3.888222630716485107E-17, -0.9482591181445367834 ) ) ;
#17907=DIRECTION ( 'NONE',  ( 0.000000000000000000, 0.000000000000000000, -1.000000000000000000 ) ) ;
#17911=DIRECTION ( 'NONE',  ( -1.000000000000000000, 0.000000000000000000, 0.000000000000000000 ) ) ;
#17919=AXIS2_PLACEMENT_3D ( 'NONE', #21792, #13309, #2429 ) ;
#17925=ADVANCED_FACE ( 'NONE', ( #23025 ), #8939, .T. ) ;
#17936=DIRECTION ( 'NONE',  ( 0.000000000000000000, 0.000000000000000000, -1.000000000000000000 ) ) ;
#17966=CARTESIAN_POINT ( 'NONE',  ( -0.5182863655200992126, 0.000000000000000000, -0.2204724409448818867 ) ) ;
#17977=ADVANCED_FACE ( 'NONE', ( #19621 ), #27004, .F. ) ;
#17980=ADVANCED_FACE ( 'NONE', ( #23988 ), #16638, .T. ) ;
#18005=DIRECTION ( 'NONE',  ( 0.8176200022776350940, 1.001295718708157488E-16, -0.5757582234545329802 ) ) ;
#18051=CARTESIAN_POINT ( 'NONE',  ( 0.000000000000000000, 0.000000000000000000, -4.370956692913385731E-17 ) ) ;
#18098=FACE_OUTER_BOUND ( 'NONE', #23263, .T. ) ;
#18155=ORIENTED_EDGE ( 'NONE', *, *, #24024, .T. ) ;
#18169=( NAMED_UNIT ( * ) PLANE_ANGLE_UNIT ( ) SI_UNIT ( $, .RADIAN. ) ) ;
#18274=ORIENTED_EDGE ( 'NONE', *, *, #3993, .F. ) ;
#18285=EDGE_CURVE ( 'NONE', #18599, #2223, #4480, .T. ) ;
#18396=CARTESIAN_POINT ( 'NONE',  ( -0.6456692913385827515, 0.000000000000000000, -0.01377952755905511792 ) ) ;
#18419=ORIENTED_EDGE ( 'NONE', *, *, #4573, .T. ) ;
#18454=ORIENTED_EDGE ( 'NONE', *, *, #2432, .F. ) ;
#18469=AXIS2_PLACEMENT_3D ( 'NONE', #16572, #18677, #6273 ) ;
#18529=DIRECTION ( 'NONE',  ( 1.000000000000000000, 0.000000000000000000, 0.000000000000000000 ) ) ;
#18579=DIRECTION ( 'NONE',  ( 0.000000000000000000, 0.000000000000000000, -1.000000000000000000 ) ) ;
#18597=VERTEX_POINT ( 'NONE', #24407 ) ;
#18599=VERTEX_POINT ( 'NONE', #4642 ) ;
#18655=VECTOR ( 'NONE', #5838, 39.37007874015748143 ) ;
#18677=DIRECTION ( 'NONE',  ( 0.000000000000000000, 0.000000000000000000, -1.000000000000000000 ) ) ;
#18686=DIRECTION ( 'NONE',  ( -1.000000000000000000, -1.224646799147353454E-16, 0.000000000000000000 ) ) ;
#18692=VERTEX_POINT ( 'NONE', #1257 ) ;
#18704=ORIENTED_EDGE ( 'NONE', *, *, #3008, .T. ) ;
#18732=FACE_OUTER_BOUND ( 'NONE', #3910, .T. ) ;
#18761=FACE_OUTER_BOUND ( 'NONE', #21028, .T. ) ;
#18800=AXIS2_PLACEMENT_3D ( 'NONE', #14082, #24806, #26788 ) ;
#18802=EDGE_CURVE ( 'NONE', #25409, #4552, #7069, .T. ) ;
#18834=AXIS2_PLACEMENT_3D ( 'NONE', #1129, #11850, #16102 ) ;
#18850=EDGE_LOOP ( 'NONE', ( #15353, #9945, #13549, #5144 ) ) ;
#18927=CARTESIAN_POINT ( 'NONE',  ( 0.000000000000000000, 0.000000000000000000, -0.1111195235210984261 ) ) ;
#18931=CARTESIAN_POINT ( 'NONE',  ( 0.000000000000000000, 0.000000000000000000, -0.1309055118110236116 ) ) ;
#18940=ORIENTED_EDGE ( 'NONE', *, *, #17078, .F. ) ;
#19022=VERTEX_POINT ( 'NONE', #4538 ) ;
#19067=EDGE_LOOP ( 'NONE', ( #13722, #15867, #15492, #3780 ) ) ;
#19104=CARTESIAN_POINT ( 'NONE',  ( 0.000000000000000000, -5.394653543307086438E-17, -0.1627508102905848297 ) ) ;
#19144=ORIENTED_EDGE ( 'NONE', *, *, #3504, .F. ) ;
#19199=ADVANCED_FACE ( 'NONE', ( #26520 ), #24218, .F. ) ;
#19303=EDGE_LOOP ( 'NONE', ( #9607, #8588, #19585, #9459 ) ) ;
#19304=CARTESIAN_POINT ( 'NONE',  ( 0.000000000000000000, 0.000000000000000000, -0.1756889763779527769 ) ) ;
#19325=ORIENTED_EDGE ( 'NONE', *, *, #14418, .T. ) ;
#19329=DIRECTION ( 'NONE',  ( 0.000000000000000000, 0.000000000000000000, -1.000000000000000000 ) ) ;
#19330=CARTESIAN_POINT ( 'NONE',  ( 0.000000000000000000, 0.000000000000000000, -0.01377952755905511792 ) ) ;
#19402=AXIS2_PLACEMENT_3D ( 'NONE', #20755, #7904, #25410 ) ;
#19417=CIRCLE ( 'NONE', #14947, 0.4986013261500205074 ) ;
#19521=EDGE_CURVE ( 'NONE', #2487, #22124, #14749, .T. ) ;
#19531=EDGE_CURVE ( 'NONE', #25409, #10563, #6171, .T. ) ;
#19536=ORIENTED_EDGE ( 'NONE', *, *, #24552, .F. ) ;
#19541=CARTESIAN_POINT ( 'NONE',  ( -0.4626586504047134341, 0.000000000000000000, -0.2204724409448818867 ) ) ;
#19551=CARTESIAN_POINT ( 'NONE',  ( 0.4986013261500205074, 6.106105181202481056E-17, -0.1756889763779527769 ) ) ;
#19561=DIRECTION ( 'NONE',  ( -1.224646799147353207E-16, 1.000000000000000000, 0.000000000000000000 ) ) ;
#19585=ORIENTED_EDGE ( 'NONE', *, *, #7479, .F. ) ;
#19618=AXIS2_PLACEMENT_3D ( 'NONE', #18051, #15971, #3366 ) ;
#19621=FACE_OUTER_BOUND ( 'NONE', #15393, .T. ) ;
#19633=DIRECTION ( 'NONE',  ( 0.000000000000000000, 0.000000000000000000, 1.000000000000000000 ) ) ;
#19661=DIRECTION ( 'NONE',  ( -1.000000000000000000, 0.000000000000000000, 0.000000000000000000 ) ) ;
#19673=CARTESIAN_POINT ( 'NONE',  ( 0.5379714048901780288, 6.588249590315613132E-17, -0.2342519685039370358 ) ) ;
#19698=DIRECTION ( 'NONE',  ( -1.000000000000000000, -1.224646799147356165E-16, 0.000000000000000000 ) ) ;
#19728=EDGE_CURVE ( 'NONE', #27804, #13542, #23307, .T. ) ;
#19749=COLOUR_RGB ( '', 0.66274510, 0.83137255, 0.94901961) ;
#19758=AXIS2_PLACEMENT_3D ( 'NONE', #1678, #3644, #16945 ) ;
#19792=DIRECTION ( 'NONE',  ( 1.000000000000000000, 0.000000000000000000, 0.000000000000000000 ) ) ;
#19842=AXIS2_PLACEMENT_3D ( 'NONE', #17457, #24224, #15364 ) ;
#19857=ORIENTED_EDGE ( 'NONE', *, *, #14605, .F. ) ;
#19872=ORIENTED_EDGE ( 'NONE', *, *, #13241, .F. ) ;
#20013=SHAPE_REPRESENTATION ( 'Shaft Seal 20x35x7', ( #11588 ), #9813 ) ;
#20031=AXIS2_PLACEMENT_3D ( 'NONE', #3989, #26689, #19792 ) ;
#20034=ORIENTED_EDGE ( 'NONE', *, *, #24999, .T. ) ;
#20083=EDGE_LOOP ( 'NONE', ( #10096, #9748 ) ) ;
#20171=ORIENTED_EDGE ( 'NONE', *, *, #55, .F. ) ;
#20172=EDGE_CURVE ( 'NONE', #10563, #18599, #1641, .T. ) ;
#20181=EDGE_CURVE ( 'NONE', #27011, #23082, #27813, .T. ) ;
#20196=DIRECTION ( 'NONE',  ( -1.000000000000000000, 0.000000000000000000, 0.000000000000000000 ) ) ;
#20240=CARTESIAN_POINT ( 'NONE',  ( 0.000000000000000000, 0.000000000000000000, -0.2480314960629921295 ) ) ;
#20276=EDGE_LOOP ( 'NONE', ( #25998, #16970, #22909, #10906 ) ) ;
#20283=EDGE_CURVE ( 'NONE', #12499, #18597, #22029, .T. ) ;
#20295=CARTESIAN_POINT ( 'NONE',  ( 0.4307823082429378392, 5.275561749190223172E-17, -0.1559029880880275776 ) ) ;
#20376=CARTESIAN_POINT ( 'NONE',  ( 0.6299212598425196763, 7.714310545810098438E-17, -0.006889763779527558960 ) ) ;
#20417=AXIS2_PLACEMENT_3D ( 'NONE', #7976, #25195, #25058 ) ;
#20431=CARTESIAN_POINT ( 'NONE',  ( 0.4986013261500205074, 6.106105181202481056E-17, -0.2204724409448818867 ) ) ;
#20449=AXIS2_PLACEMENT_3D ( 'NONE', #2267, #24160, #15295 ) ;
#20455=EDGE_LOOP ( 'NONE', ( #3548, #25498 ) ) ;
#20499=VERTEX_POINT ( 'NONE', #12582 ) ;
#20611=EDGE_CURVE ( 'NONE', #25295, #13542, #24278, .T. ) ;
#20617=PRODUCT_DEFINITION_SHAPE ( 'NONE', 'NONE',  #23987 ) ;
#20618=EDGE_CURVE ( 'NONE', #15239, #21578, #14288, .T. ) ;
#20667=TOROIDAL_SURFACE ( 'NONE', #18800, 0.6751968503937006982, 0.01377952755905511792 ) ;
#20669=DIRECTION ( 'NONE',  ( 0.000000000000000000, 0.000000000000000000, 1.000000000000000000 ) ) ;
#20683=CARTESIAN_POINT ( 'NONE',  ( 0.4986013261500205074, 6.106105181202481056E-17, -0.1033464566929133965 ) ) ;
#20723=DIRECTION ( 'NONE',  ( 0.000000000000000000, 0.000000000000000000, -1.000000000000000000 ) ) ;
#20755=CARTESIAN_POINT ( 'NONE',  ( -0.4325730547867440712, 0.000000000000000000, -0.1740172276534823204 ) ) ;
#20768=EDGE_CURVE ( 'NONE', #2223, #18599, #24736, .T. ) ;
#20807=ORIENTED_EDGE ( 'NONE', *, *, #6186, .F. ) ;
#20820=SURFACE_SIDE_STYLE ('',( #16314 ) ) ;
#20901=UNCERTAINTY_MEASURE_WITH_UNIT (LENGTH_MEASURE( 1.000000000000000082E-05 ), #1336, 'distance_accuracy_value', 'NONE') ;
#20919=DIRECTION ( 'NONE',  ( -1.000000000000000000, 0.000000000000000000, 0.000000000000000000 ) ) ;
#20943=ORIENTED_EDGE ( 'NONE', *, *, #22676, .T. ) ;
#20966=( NAMED_UNIT ( * ) SI_UNIT ( $, .STERADIAN. ) SOLID_ANGLE_UNIT ( ) ) ;
#20972=CIRCLE ( 'NONE', #17368, 0.4986013261500205074 ) ;
#20992=DIRECTION ( 'NONE',  ( 0.000000000000000000, 0.000000000000000000, -1.000000000000000000 ) ) ;
#21028=EDGE_LOOP ( 'NONE', ( #15993, #27708, #16651, #19144 ) ) ;
#21087=DIRECTION ( 'NONE',  ( 0.000000000000000000, 0.000000000000000000, -1.000000000000000000 ) ) ;
#21170=DIRECTION ( 'NONE',  ( -0.3174974722037089969, 0.000000000000000000, -0.9482591181445370054 ) ) ;
#21202=ORIENTED_EDGE ( 'NONE', *, *, #8676, .F. ) ;
#21225=ADVANCED_FACE ( 'NONE', ( #3558 ), #12189, .T. ) ;
#21278=DIRECTION ( 'NONE',  ( 0.000000000000000000, 0.000000000000000000, -1.000000000000000000 ) ) ;
#21287=FACE_OUTER_BOUND ( 'NONE', #16889, .T. ) ;
#21325=AXIS2_PLACEMENT_3D ( 'NONE', #14440, #16830, #20919 ) ;
#21401=DIRECTION ( 'NONE',  ( 0.000000000000000000, 0.000000000000000000, -1.000000000000000000 ) ) ;
#21403=AXIS2_PLACEMENT_3D ( 'NONE', #14536, #23429, #1792 ) ;
#21406=CARTESIAN_POINT ( 'NONE',  ( 0.6889763779527560139, 8.437527159479796553E-17, -0.1377952755905511861 ) ) ;
#21462=DIRECTION ( 'NONE',  ( 1.000000000000000000, 0.000000000000000000, 0.000000000000000000 ) ) ;
#21525=DIRECTION ( 'NONE',  ( 0.000000000000000000, 0.000000000000000000, -1.000000000000000000 ) ) ;
#21578=VERTEX_POINT ( 'NONE', #4390 ) ;
#21596=AXIS2_PLACEMENT_3D ( 'NONE', #17132, #9054, #25753 ) ;
#21619=CARTESIAN_POINT ( 'NONE',  ( -0.4848217985909654137, 0.000000000000000000, -0.05511811023622047168 ) ) ;
#21628=AXIS2_PLACEMENT_3D ( 'NONE', #24811, #20723, #25096 ) ;
#21671=AXIS2_PLACEMENT_3D ( 'NONE', #15835, #22335, #2962 ) ;
#21673=DIRECTION ( 'NONE',  ( 0.000000000000000000, 0.000000000000000000, -1.000000000000000000 ) ) ;
#21682=EDGE_CURVE ( 'NONE', #13237, #16707, #1863, .T. ) ;
#21693=DIRECTION ( 'NONE',  ( -0.000000000000000000, -1.000000000000000000, -0.000000000000000000 ) ) ;
#21700=CARTESIAN_POINT ( 'NONE',  ( 0.6751968503937006982, 8.268776616290199217E-17, -0.01377952755905511792 ) ) ;
#21747=AXIS2_PLACEMENT_3D ( 'NONE', #15734, #13883, #22218 ) ;
#21756=CARTESIAN_POINT ( 'NONE',  ( 0.000000000000000000, 0.000000000000000000, -0.1559029880880275776 ) ) ;
#21772=DIRECTION ( 'NONE',  ( 0.000000000000000000, 0.000000000000000000, -1.000000000000000000 ) ) ;
#21792=CARTESIAN_POINT ( 'NONE',  ( 0.000000000000000000, 0.000000000000000000, -0.1377952755905511861 ) ) ;
#21796=CIRCLE ( 'NONE', #23160, 0.01377952755905510404 ) ;
#21803=ADVANCED_FACE ( 'NONE', ( #23840 ), #8634, .F. ) ;
#21838=EDGE_CURVE ( 'NONE', #4552, #25079, #15226, .T. ) ;
#21848=CYLINDRICAL_SURFACE ( 'NONE', #11149, 0.6614173228346456046 ) ;
#21884=AXIS2_PLACEMENT_3D ( 'NONE', #19304, #363, #7778 ) ;
#21916=EDGE_CURVE ( 'NONE', #16707, #13237, #17469, .T. ) ;
#21963=CARTESIAN_POINT ( 'NONE',  ( 0.000000000000000000, 0.000000000000000000, -0.01377952755905511792 ) ) ;
#21974=ORIENTED_EDGE ( 'NONE', *, *, #12795, .T. ) ;
#21978=ORIENTED_EDGE ( 'NONE', *, *, #20768, .F. ) ;
#21992=FACE_OUTER_BOUND ( 'NONE', #23724, .T. ) ;
#21995=ORIENTED_EDGE ( 'NONE', *, *, #8917, .F. ) ;
#22029=CIRCLE ( 'NONE', #21596, 0.5379714048901780288 ) ;
#22083=DIRECTION ( 'NONE',  ( 1.000000000000000000, 0.000000000000000000, 0.000000000000000000 ) ) ;
#22097=CARTESIAN_POINT ( 'NONE',  ( -0.6751968503937006982, 0.000000000000000000, -0.01377952755905511792 ) ) ;
#22098=ADVANCED_FACE ( 'NONE', ( #26046 ), #6232, .F. ) ;
#22101=ADVANCED_FACE ( 'NONE', ( #2184, #12775 ), #12912, .T. ) ;
#22124=VERTEX_POINT ( 'NONE', #14925 ) ;
#22128=ADVANCED_FACE ( 'NONE', ( #2579 ), #24068, .F. ) ;
#22150=AXIS2_PLACEMENT_3D ( 'NONE', #17042, #14940, #12654 ) ;
#22191=ORIENTED_EDGE ( 'NONE', *, *, #25846, .T. ) ;
#22215=DIRECTION ( 'NONE',  ( -1.000000000000000000, 0.000000000000000000, 0.000000000000000000 ) ) ;
#22218=DIRECTION ( 'NONE',  ( -1.000000000000000000, 0.000000000000000000, 0.000000000000000000 ) ) ;
#22263=ORIENTED_EDGE ( 'NONE', *, *, #4573, .F. ) ;
#22335=DIRECTION ( 'NONE',  ( 0.000000000000000000, 0.000000000000000000, -1.000000000000000000 ) ) ;
#22356=EDGE_CURVE ( 'NONE', #16402, #25917, #25710, .T. ) ;
#22358=ADVANCED_FACE ( 'NONE', ( #1838 ), #12045, .T. ) ;
#22443=EDGE_LOOP ( 'NONE', ( #19872, #20034, #7218, #11332 ) ) ;
#22446=DIRECTION ( 'NONE',  ( -1.000000000000000000, 0.000000000000000000, 0.000000000000000000 ) ) ;
#22510=EDGE_LOOP ( 'NONE', ( #24968, #27403, #22191, #16899 ) ) ;
#22666=( LENGTH_UNIT ( ) NAMED_UNIT ( * ) SI_UNIT ( $, .METRE. ) ) ;
#22671=ORIENTED_EDGE ( 'NONE', *, *, #23404, .F. ) ;
#22676=EDGE_CURVE ( 'NONE', #4895, #12340, #11424, .T. ) ;
#22695=DIRECTION ( 'NONE',  ( 1.000000000000000000, 0.000000000000000000, 0.000000000000000000 ) ) ;
#22775=TOROIDAL_SURFACE ( 'NONE', #9223, 0.4986013261500205074, 0.02755905511811023584 ) ;
#22820=CARTESIAN_POINT ( 'NONE',  ( -0.4986013261500205074, 0.000000000000000000, -0.05511811023622047168 ) ) ;
#22869=DIRECTION ( 'NONE',  ( 0.000000000000000000, 0.000000000000000000, 1.000000000000000000 ) ) ;
#22889=CARTESIAN_POINT ( 'NONE',  ( -0.5241918773311228241, 0.000000000000000000, -0.2342519685039370358 ) ) ;
#22909=ORIENTED_EDGE ( 'NONE', *, *, #18802, .T. ) ;
#22925=LINE ( 'NONE', #20376, #18655 ) ;
#22950=CYLINDRICAL_SURFACE ( 'NONE', #24140, 0.5379714048901780288 ) ;
#22952=DIRECTION ( 'NONE',  ( -1.224646799147353207E-16, 1.000000000000000000, 0.000000000000000000 ) ) ;
#22964=FACE_OUTER_BOUND ( 'NONE', #4476, .T. ) ;
#23004=SHAPE_DEFINITION_REPRESENTATION ( #20617, #20013 ) ;
#23025=FACE_OUTER_BOUND ( 'NONE', #20276, .T. ) ;
#23039=VERTEX_POINT ( 'NONE', #20431 ) ;
#23052=VERTEX_POINT ( 'NONE', #11669 ) ;
#23082=VERTEX_POINT ( 'NONE', #2056 ) ;
#23094=PRESENTATION_STYLE_ASSIGNMENT (( #14053 ) ) ;
#23099=CIRCLE ( 'NONE', #24892, 0.5241918773311228241 ) ;
#23130=DIRECTION ( 'NONE',  ( 0.000000000000000000, 0.000000000000000000, -1.000000000000000000 ) ) ;
#23160=AXIS2_PLACEMENT_3D ( 'NONE', #1697, #25713, #5809 ) ;
#23211=CIRCLE ( 'NONE', #13252, 0.5241918773311228241 ) ;
#23263=EDGE_LOOP ( 'NONE', ( #8213, #18155 ) ) ;
#23272=VECTOR ( 'NONE', #17672, 39.37007874015748143 ) ;
#23303=LINE ( 'NONE', #3930, #14569 ) ;
#23307=CIRCLE ( 'NONE', #9256, 0.02755905511811023931 ) ;
#23338=DIRECTION ( 'NONE',  ( -1.000000000000000000, 0.000000000000000000, 0.000000000000000000 ) ) ;
#23366=ORIENTED_EDGE ( 'NONE', *, *, #12420, .F. ) ;
#23384=ORIENTED_EDGE ( 'NONE', *, *, #24999, .F. ) ;
#23393=MECHANICAL_DESIGN_GEOMETRIC_PRESENTATION_REPRESENTATION('',(#16571),#8499);
#23404=EDGE_CURVE ( 'NONE', #12651, #25917, #15954, .T. ) ;
#23429=DIRECTION ( 'NONE',  ( -1.224646799147353207E-16, 1.000000000000000000, 0.000000000000000000 ) ) ;
#23444=EDGE_CURVE ( 'NONE', #27804, #23052, #13227, .T. ) ;
#23472=DIRECTION ( 'NONE',  ( 0.000000000000000000, 0.000000000000000000, -1.000000000000000000 ) ) ;
#23495=AXIS2_PLACEMENT_3D ( 'NONE', #12479, #6410, #23517 ) ;
#23503=CARTESIAN_POINT ( 'NONE',  ( 0.5241918773311228241, 6.503874318720813848E-17, -0.2204724409448818867 ) ) ;
#23517=DIRECTION ( 'NONE',  ( -1.000000000000000000, 0.000000000000000000, 0.000000000000000000 ) ) ;
#23534=CARTESIAN_POINT ( 'NONE',  ( 0.000000000000000000, 0.000000000000000000, -0.1309055118110236116 ) ) ;
#23650=ORIENTED_EDGE ( 'NONE', *, *, #8676, .T. ) ;
#23675=VECTOR ( 'NONE', #18005, 39.37007874015748854 ) ;
#23724=EDGE_LOOP ( 'NONE', ( #19857, #5055, #25687, #6322 ) ) ;
#23740=ORIENTED_EDGE ( 'NONE', *, *, #24541, .T. ) ;
#23741=CARTESIAN_POINT ( 'NONE',  ( 0.000000000000000000, 0.000000000000000000, -0.1756889763779527769 ) ) ;
#23784=EDGE_CURVE ( 'NONE', #11118, #12651, #12973, .T. ) ;
#23789=LINE ( 'NONE', #25902, #26301 ) ;
#23828=ORIENTED_EDGE ( 'NONE', *, *, #24514, .F. ) ;
#23834=CYLINDRICAL_SURFACE ( 'NONE', #21884, 0.4986013261500205074 ) ;
#23840=FACE_OUTER_BOUND ( 'NONE', #1214, .T. ) ;
#23872=DIRECTION ( 'NONE',  ( 0.000000000000000000, 0.000000000000000000, 1.000000000000000000 ) ) ;
#23889=ORIENTED_EDGE ( 'NONE', *, *, #20618, .F. ) ;
#23896=DIRECTION ( 'NONE',  ( 0.000000000000000000, 0.000000000000000000, -1.000000000000000000 ) ) ;
#23924=CIRCLE ( 'NONE', #18469, 0.3937007874015748254 ) ;
#23960=EDGE_CURVE ( 'NONE', #11811, #12052, #23211, .T. ) ;
#23987=PRODUCT_DEFINITION ( 'UNKNOWN', '', #5786, #6282 ) ;
#23988=FACE_OUTER_BOUND ( 'NONE', #12017, .T. ) ;
#23998=CARTESIAN_POINT ( 'NONE',  ( -0.4616918773311228796, 0.000000000000000000, -0.04133858267716535029 ) ) ;
#24024=EDGE_CURVE ( 'NONE', #16539, #26492, #1541, .T. ) ;
#24068=CYLINDRICAL_SURFACE ( 'NONE', #25148, 0.6614173228346456046 ) ;
#24076=EDGE_LOOP ( 'NONE', ( #16928, #21974, #5235, #17019 ) ) ;
#24102=ORIENTED_EDGE ( 'NONE', *, *, #13853, .F. ) ;
#24109=VERTEX_POINT ( 'NONE', #24704 ) ;
#24113=ORIENTED_EDGE ( 'NONE', *, *, #15114, .T. ) ;
#24140=AXIS2_PLACEMENT_3D ( 'NONE', #3565, #12066, #10078 ) ;
#24160=DIRECTION ( 'NONE',  ( 0.000000000000000000, 0.000000000000000000, -1.000000000000000000 ) ) ;
#24186=AXIS2_PLACEMENT_3D ( 'NONE', #15170, #15316, #4138 ) ;
#24190=DIRECTION ( 'NONE',  ( -0.3174974722037094410, 0.000000000000000000, -0.9482591181445367834 ) ) ;
#24193=CARTESIAN_POINT ( 'NONE',  ( 0.4405067310592692409, 5.394651581945980194E-17, -0.1627508102905848297 ) ) ;
#24212=DIRECTION ( 'NONE',  ( 1.000000000000000000, 0.000000000000000000, 0.000000000000000000 ) ) ;
#24218=CONICAL_SURFACE ( 'NONE', #7087, 0.4307823082429378392, 0.9572651268756555698 ) ;
#24224=DIRECTION ( 'NONE',  ( 0.000000000000000000, 0.000000000000000000, -1.000000000000000000 ) ) ;
#24242=DIRECTION ( 'NONE',  ( -1.000000000000000000, 0.000000000000000000, 0.000000000000000000 ) ) ;
#24270=TOROIDAL_SURFACE ( 'NONE', #27431, 0.5241918773311228241, 0.01377952755905511792 ) ;
#24278=CIRCLE ( 'NONE', #12103, 0.4986013261500205074 ) ;
#24279=VERTEX_POINT ( 'NONE', #19673 ) ;
#24307=CARTESIAN_POINT ( 'NONE',  ( -0.6614173228346456046, 0.000000000000000000, -0.01377952755905511792 ) ) ;
#24334=DIRECTION ( 'NONE',  ( 0.000000000000000000, 0.000000000000000000, -1.000000000000000000 ) ) ;
#24352=DIRECTION ( 'NONE',  ( 0.000000000000000000, 0.000000000000000000, -1.000000000000000000 ) ) ;
#24407=CARTESIAN_POINT ( 'NONE',  ( -0.5379714048901780288, 0.000000000000000000, -0.2480314960629921295 ) ) ;
#24514=EDGE_CURVE ( 'NONE', #26492, #16539, #26816, .T. ) ;
#24524=LINE ( 'NONE', #20295, #23675 ) ;
#24541=EDGE_CURVE ( 'NONE', #15200, #3726, #17354, .T. ) ;
#24547=AXIS2_PLACEMENT_3D ( 'NONE', #19104, #20669, #18529 ) ;
#24552=EDGE_CURVE ( 'NONE', #24279, #24109, #5145, .T. ) ;
#24556=PLANE ( 'NONE',  #18834 ) ;
#24615=ORIENTED_EDGE ( 'NONE', *, *, #10010, .F. ) ;
#24687=CIRCLE ( 'NONE', #16140, 0.02755905511811020808 ) ;
#24704=CARTESIAN_POINT ( 'NONE',  ( -0.5379714048901780288, 0.000000000000000000, -0.2342519685039370358 ) ) ;
#24734=DIRECTION ( 'NONE',  ( 0.000000000000000000, 0.000000000000000000, -1.000000000000000000 ) ) ;
#24736=CIRCLE ( 'NONE', #4470, 0.6751968503937006982 ) ;
#24748=CONICAL_SURFACE ( 'NONE', #26534, 0.4092416079569000109, 0.7340599135827593491 ) ;
#24766=DIRECTION ( 'NONE',  ( 0.000000000000000000, 0.000000000000000000, 1.000000000000000000 ) ) ;
#24806=DIRECTION ( 'NONE',  ( 0.000000000000000000, 0.000000000000000000, -1.000000000000000000 ) ) ;
#24810=CONICAL_SURFACE ( 'NONE', #3143, 0.4626586504047134341, 0.3230892413134545116 ) ;
#24811=CARTESIAN_POINT ( 'NONE',  ( 0.000000000000000000, -5.457511811023621697E-17, -0.1696422624804970747 ) ) ;
#24841=ORIENTED_EDGE ( 'NONE', *, *, #20172, .T. ) ;
#24892=AXIS2_PLACEMENT_3D ( 'NONE', #3382, #14155, #27425 ) ;
#24968=ORIENTED_EDGE ( 'NONE', *, *, #24024, .F. ) ;
#24979=ORIENTED_EDGE ( 'NONE', *, *, #17069, .T. ) ;
#24983=AXIS2_PLACEMENT_3D ( 'NONE', #9588, #26982, #20196 ) ;
#24990=DIRECTION ( 'NONE',  ( 0.000000000000000000, 0.000000000000000000, -1.000000000000000000 ) ) ;
#24999=EDGE_CURVE ( 'NONE', #19022, #3726, #24524, .T. ) ;
#25002=ORIENTED_EDGE ( 'NONE', *, *, #6905, .T. ) ;
#25058=DIRECTION ( 'NONE',  ( -1.000000000000000000, 0.000000000000000000, 0.000000000000000000 ) ) ;
#25059=LENGTH_MEASURE_WITH_UNIT ( LENGTH_MEASURE( 0.02539999999999999897 ), #22666 ) ;
#25079=VERTEX_POINT ( 'NONE', #3467 ) ;
#25096=DIRECTION ( 'NONE',  ( 1.000000000000000000, 0.000000000000000000, 0.000000000000000000 ) ) ;
#25148=AXIS2_PLACEMENT_3D ( 'NONE', #23534, #21401, #17160 ) ;
#25160=DIRECTION ( 'NONE',  ( -1.000000000000000000, 0.000000000000000000, 0.000000000000000000 ) ) ;
#25195=DIRECTION ( 'NONE',  ( 0.000000000000000000, 0.000000000000000000, 1.000000000000000000 ) ) ;
#25205=ORIENTED_EDGE ( 'NONE', *, *, #18285, .F. ) ;
#25234=CYLINDRICAL_SURFACE ( 'NONE', #17794, 0.4986013261500205074 ) ;
#25238=ADVANCED_FACE ( 'NONE', ( #21287 ), #25234, .T. ) ;
#25295=VERTEX_POINT ( 'NONE', #15624 ) ;
#25339=FILL_AREA_STYLE ('',( #12346 ) ) ;
#25341=VECTOR ( 'NONE', #13137, 39.37007874015748143 ) ;
#25381=CARTESIAN_POINT ( 'NONE',  ( 0.000000000000000000, 0.000000000000000000, -0.1377952755905511861 ) ) ;
#25409=VERTEX_POINT ( 'NONE', #9615 ) ;
#25410=DIRECTION ( 'NONE',  ( 0.000000000000000000, 0.000000000000000000, -1.000000000000000000 ) ) ;
#25430=DIRECTION ( 'NONE',  ( 1.000000000000000000, 0.000000000000000000, 0.000000000000000000 ) ) ;
#25463=ADVANCED_FACE ( 'NONE', ( #1574 ), #4287, .T. ) ;
#25464=FACE_OUTER_BOUND ( 'NONE', #13485, .T. ) ;
#25498=ORIENTED_EDGE ( 'NONE', *, *, #25846, .F. ) ;
#25557=CARTESIAN_POINT ( 'NONE',  ( 0.000000000000000000, 0.000000000000000000, -0.2204724409448818867 ) ) ;
#25667=DIRECTION ( 'NONE',  ( -1.000000000000000000, 0.000000000000000000, 0.000000000000000000 ) ) ;
#25687=ORIENTED_EDGE ( 'NONE', *, *, #13018, .T. ) ;
#25698=TOROIDAL_SURFACE ( 'NONE', #19842, 0.4325730547867440712, 0.01377952755905511792 ) ;
#25710=LINE ( 'NONE', #6362, #1337 ) ;
#25713=DIRECTION ( 'NONE',  ( -1.224646799147353207E-16, 1.000000000000000000, 0.000000000000000000 ) ) ;
#25724=EDGE_LOOP ( 'NONE', ( #2548, #23828, #13979, #4345 ) ) ;
#25726=TOROIDAL_SURFACE ( 'NONE', #21671, 0.6751968503937006982, 0.01377952755905511792 ) ;
#25730=FACE_OUTER_BOUND ( 'NONE', #19067, .T. ) ;
#25753=DIRECTION ( 'NONE',  ( -1.000000000000000000, 0.000000000000000000, 0.000000000000000000 ) ) ;
#25831=EDGE_LOOP ( 'NONE', ( #26621, #24979, #14506, #22671 ) ) ;
#25833=CARTESIAN_POINT ( 'NONE',  ( 0.000000000000000000, 0.000000000000000000, -0.1111195235210984261 ) ) ;
#25846=EDGE_CURVE ( 'NONE', #22124, #2487, #2923, .T. ) ;
#25878=AXIS2_PLACEMENT_3D ( 'NONE', #9326, #17936, #1020 ) ;
#25894=CLOSED_SHELL ( 'NONE', ( #12995, #10258, #12600, #25238, #21803, #7043, #7657, #25463, #21225, #17925, #5488, #11352, #5239, #17980, #15643, #27841, #17008, #22128, #5353, #22358, #1182, #9692, #17977, #10649, #22101, #16384, #17663, #2604, #3097, #19199, #22098, #6521, #11884, #12088, #17797, #26005, #8310, #3205 ) ) ;
#25902=CARTESIAN_POINT ( 'NONE',  ( -0.4986013261500205074, 0.000000000000000000, -0.05856299212598425896 ) ) ;
#25916=DIRECTION ( 'NONE',  ( 0.000000000000000000, 0.000000000000000000, 1.000000000000000000 ) ) ;
#25917=VERTEX_POINT ( 'NONE', #12863 ) ;
#25998=ORIENTED_EDGE ( 'NONE', *, *, #14761, .T. ) ;
#26005=ADVANCED_FACE ( 'NONE', ( #25730 ), #22950, .T. ) ;
#26046=FACE_OUTER_BOUND ( 'NONE', #9954, .T. ) ;
#26059=ORIENTED_EDGE ( 'NONE', *, *, #10547, .F. ) ;
#26099=CIRCLE ( 'NONE', #13916, 0.4173606904906118076 ) ;
#26104=CARTESIAN_POINT ( 'NONE',  ( 0.4986013261500205074, 6.106105181202481056E-17, -0.05856299212598425896 ) ) ;
#26109=EDGE_LOOP ( 'NONE', ( #15309, #11257, #12512, #4062 ) ) ;
#26110=DIRECTION ( 'NONE',  ( 0.6698894744055998718, -8.203780006133206145E-17, 0.7424608353849979636 ) ) ;
#26118=FACE_BOUND ( 'NONE', #6539, .T. ) ;
#26137=CIRCLE ( 'NONE', #21628, 0.4456396174367268093 ) ;
#26225=CYLINDRICAL_SURFACE ( 'NONE', #15025, 0.6299212598425196763 ) ;
#26236=AXIS2_PLACEMENT_3D ( 'NONE', #27623, #10092, #7989 ) ;
#26301=VECTOR ( 'NONE', #15178, 39.37007874015748143 ) ;
#26329=EDGE_LOOP ( 'NONE', ( #26873, #14835, #6765, #8082 ) ) ;
#26343=CARTESIAN_POINT ( 'NONE',  ( 0.000000000000000000, 0.000000000000000000, -0.1464516454673935042 ) ) ;
#26402=DIRECTION ( 'NONE',  ( 0.000000000000000000, 0.000000000000000000, -1.000000000000000000 ) ) ;
#26415=AXIS2_PLACEMENT_3D ( 'NONE', #10938, #19561, #19698 ) ;
#26417=FACE_OUTER_BOUND ( 'NONE', #19303, .T. ) ;
#26460=DIRECTION ( 'NONE',  ( 0.000000000000000000, 0.000000000000000000, -1.000000000000000000 ) ) ;
#26492=VERTEX_POINT ( 'NONE', #24307 ) ;
#26510=ADVANCED_BREP_SHAPE_REPRESENTATION ( 'Shaft Seal 20x35x7', ( #3022, #11588 ), #9813 ) ;
#26520=FACE_OUTER_BOUND ( 'NONE', #12436, .T. ) ;
#26534=AXIS2_PLACEMENT_3D ( 'NONE', #13560, #9307, #17911 ) ;
#26540=CARTESIAN_POINT ( 'NONE',  ( -0.5379714048901780288, 0.000000000000000000, -0.2342519685039370358 ) ) ;
#26547=DIRECTION ( 'NONE',  ( -1.000000000000000000, 0.000000000000000000, 0.000000000000000000 ) ) ;
#26557=CIRCLE ( 'NONE', #877, 0.3937007874015748254 ) ;
#26621=ORIENTED_EDGE ( 'NONE', *, *, #23784, .F. ) ;
#26652=DIRECTION ( 'NONE',  ( -1.000000000000000000, 0.000000000000000000, 0.000000000000000000 ) ) ;
#26672=ORIENTED_EDGE ( 'NONE', *, *, #19728, .T. ) ;
#26675=CARTESIAN_POINT ( 'NONE',  ( 0.000000000000000000, 0.000000000000000000, -0.2755905511811023723 ) ) ;
#26689=DIRECTION ( 'NONE',  ( 0.000000000000000000, 0.000000000000000000, -1.000000000000000000 ) ) ;
#26739=CIRCLE ( 'NONE', #25878, 0.4986013261500205074 ) ;
#26744=PLANE ( 'NONE',  #909 ) ;
#26788=DIRECTION ( 'NONE',  ( -1.000000000000000000, 0.000000000000000000, 0.000000000000000000 ) ) ;
#26811=LENGTH_MEASURE_WITH_UNIT ( LENGTH_MEASURE( 0.02539999999999999897 ), #17768 ) ;
#26816=CIRCLE ( 'NONE', #16437, 0.6614173228346456046 ) ;
#26822=DIRECTION ( 'NONE',  ( 0.000000000000000000, 0.000000000000000000, -1.000000000000000000 ) ) ;
#26835=DIRECTION ( 'NONE',  ( -0.000000000000000000, -1.000000000000000000, -0.000000000000000000 ) ) ;
#26870=EDGE_CURVE ( 'NONE', #27503, #12340, #26897, .T. ) ;
#26873=ORIENTED_EDGE ( 'NONE', *, *, #17069, .F. ) ;
#26897=CIRCLE ( 'NONE', #17420, 0.01377952755905511965 ) ;
#26928=AXIS2_PLACEMENT_3D ( 'NONE', #21963, #495, #24212 ) ;
#26981=LINE ( 'NONE', #26540, #1062 ) ;
#26982=DIRECTION ( 'NONE',  ( 0.000000000000000000, 0.000000000000000000, -1.000000000000000000 ) ) ;
#27004=CONICAL_SURFACE ( 'NONE', #850, 0.4055307389460929279, 0.3230892413134540120 ) ;
#27011=VERTEX_POINT ( 'NONE', #15547 ) ;
#27093=AXIS2_PLACEMENT_3D ( 'NONE', #23998, #19633, #2373 ) ;
#27097=DIRECTION ( 'NONE',  ( 0.000000000000000000, 0.000000000000000000, -1.000000000000000000 ) ) ;
#27104=ORIENTED_EDGE ( 'NONE', *, *, #12420, .T. ) ;
#27125=EDGE_CURVE ( 'NONE', #16402, #18692, #17209, .T. ) ;
#27127=ORIENTED_EDGE ( 'NONE', *, *, #9851, .F. ) ;
#27177=DIRECTION ( 'NONE',  ( 0.000000000000000000, 0.000000000000000000, 1.000000000000000000 ) ) ;
#27219=CARTESIAN_POINT ( 'NONE',  ( 0.000000000000000000, 0.000000000000000000, -0.2755905511811023723 ) ) ;
#27227=AXIS2_PLACEMENT_3D ( 'NONE', #10000, #22869, #12120 ) ;
#27237=ORIENTED_EDGE ( 'NONE', *, *, #14761, .F. ) ;
#27247=VECTOR ( 'NONE', #17823, 39.37007874015748854 ) ;
#27281=CARTESIAN_POINT ( 'NONE',  ( -0.3937007874015748254, 0.000000000000000000, -0.07578740157480315376 ) ) ;
#27340=EDGE_CURVE ( 'NONE', #14847, #4552, #7064, .T. ) ;
#27341=AXIS2_PLACEMENT_3D ( 'NONE', #25381, #12390, #25667 ) ;
#27367=CARTESIAN_POINT ( 'NONE',  ( 0.000000000000000000, 0.000000000000000000, -0.2204724409448818867 ) ) ;
#27403=ORIENTED_EDGE ( 'NONE', *, *, #8868, .T. ) ;
#27425=DIRECTION ( 'NONE',  ( 1.000000000000000000, 0.000000000000000000, 0.000000000000000000 ) ) ;
#27431=AXIS2_PLACEMENT_3D ( 'NONE', #3424, #24352, #5281 ) ;
#27503=VERTEX_POINT ( 'NONE', #16435 ) ;
#27513=CARTESIAN_POINT ( 'NONE',  ( -0.6299212598425196763, 0.000000000000000000, -0.006889763779527558960 ) ) ;
#27566=DIRECTION ( 'NONE',  ( 0.000000000000000000, 0.000000000000000000, -1.000000000000000000 ) ) ;
#27623=CARTESIAN_POINT ( 'NONE',  ( 0.000000000000000000, 0.000000000000000000, -0.05511811023622047168 ) ) ;
#27638=FACE_OUTER_BOUND ( 'NONE', #4786, .T. ) ;
#27663=AXIS2_PLACEMENT_3D ( 'NONE', #26343, #507, #15493 ) ;
#27708=ORIENTED_EDGE ( 'NONE', *, *, #55, .T. ) ;
#27804=VERTEX_POINT ( 'NONE', #11727 ) ;
#27813=CIRCLE ( 'NONE', #8856, 0.4456396174367268093 ) ;
#27820=DIRECTION ( 'NONE',  ( -1.000000000000000000, 0.000000000000000000, 0.000000000000000000 ) ) ;
#27841=ADVANCED_FACE ( 'NONE', ( #6741 ), #21848, .F. ) ;
#27846=CYLINDRICAL_SURFACE ( 'NONE', #21325, 0.5379714048901780288 ) ;
#27871=AXIS2_PLACEMENT_3D ( 'NONE', #13057, #25916, #8814 ) ;
ENDSEC;
END-ISO-10303-21;
